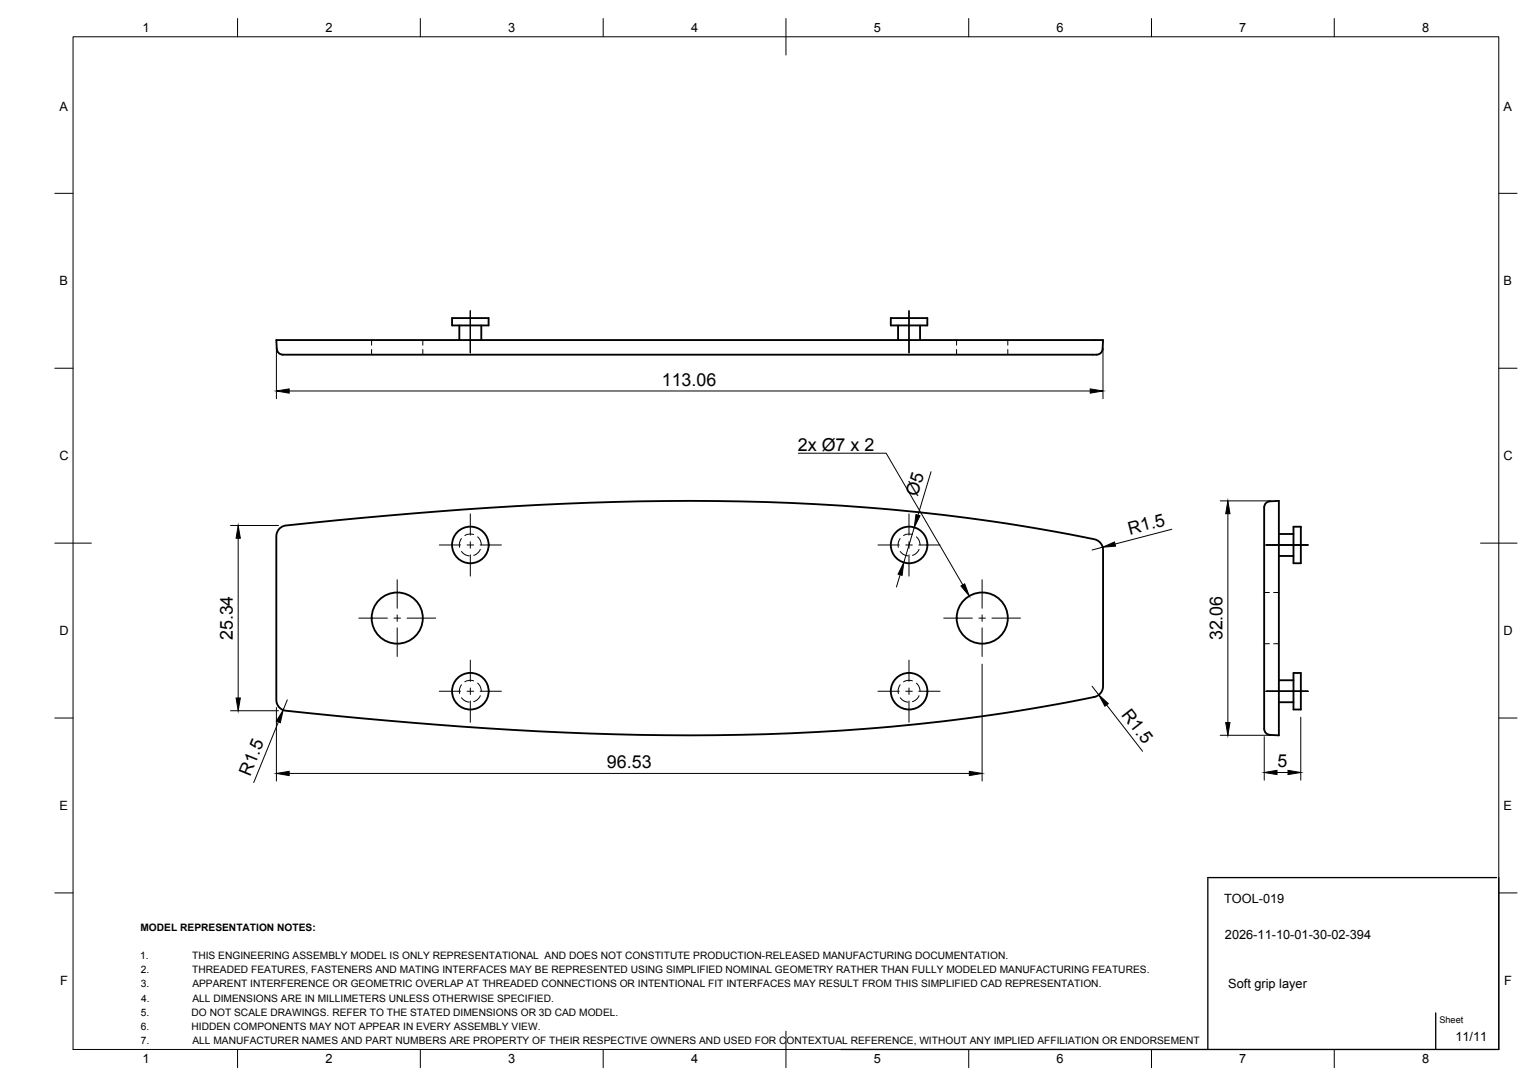
ISO-10303-21;
HEADER;
/* Generated by software containing ST-Developer
 * from STEP Tools, Inc. (www.steptools.com) 
 */

FILE_DESCRIPTION(
/* description */ (''),
/* implementation_level */ '2;1');

FILE_NAME(
/* name */ 'Soft grip layer.step',
/* time_stamp */ '2026-11-10T09:14:46-08:00',
/* author */ (''),
/* organization */ (''),
/* preprocessor_version */ 'ST-DEVELOPER v20.2',
/* originating_system */ 'Autodesk Translation Framework v15.17.0.0',
/* authorisation */ '');

FILE_SCHEMA (('AUTOMOTIVE_DESIGN { 1 0 10303 214 3 1 1 }'));
ENDSEC;

DATA;
#10=MECHANICAL_DESIGN_GEOMETRIC_PRESENTATION_REPRESENTATION('',(#564),#19471);
#156=B_SPLINE_SURFACE_WITH_KNOTS('',3,3,((#13811,#13812,#13813,#13814,#13815),
(#13816,#13817,#13818,#13819,#13820),(#13821,#13822,#13823,#13824,#13825),
(#13826,#13827,#13828,#13829,#13830),(#13831,#13832,#13833,#13834,#13835)),
 .UNSPECIFIED.,.F.,.F.,.F.,(4,1,4),(4,1,4),(0.,0.571428571428571,1.),(0.,
0.0439228984074713,0.102486762950766),.UNSPECIFIED.);
#157=B_SPLINE_SURFACE_WITH_KNOTS('',3,3,((#13858,#13859,#13860,#13861,#13862),
(#13863,#13864,#13865,#13866,#13867),(#13868,#13869,#13870,#13871,#13872),
(#13873,#13874,#13875,#13876,#13877),(#13878,#13879,#13880,#13881,#13882)),
 .UNSPECIFIED.,.F.,.F.,.F.,(4,1,4),(4,1,4),(0.,0.571428571428571,1.),(0.,
0.0439228984484775,0.102486763046448),.UNSPECIFIED.);
#158=B_SPLINE_SURFACE_WITH_KNOTS('',3,3,((#13896,#13897,#13898,#13899,#13900,
#13901),(#13902,#13903,#13904,#13905,#13906,#13907),(#13908,#13909,#13910,
#13911,#13912,#13913),(#13914,#13915,#13916,#13917,#13918,#13919),(#13920,
#13921,#13922,#13923,#13924,#13925)),.UNSPECIFIED.,.F.,.F.,.F.,(4,1,4),
(4,1,1,4),(0.,0.571428571428571,1.),(0.,4.74079765360458,7.9013294226743,
11.061861191744),.UNSPECIFIED.);
#159=B_SPLINE_SURFACE_WITH_KNOTS('',3,3,((#13941,#13942,#13943,#13944,#13945),
(#13946,#13947,#13948,#13949,#13950),(#13951,#13952,#13953,#13954,#13955),
(#13956,#13957,#13958,#13959,#13960),(#13961,#13962,#13963,#13964,#13965)),
 .UNSPECIFIED.,.F.,.F.,.F.,(4,1,4),(4,1,4),(0.,0.571428571428571,1.),(0.,
0.0409389169025732,0.0955241394393374),.UNSPECIFIED.);
#160=B_SPLINE_SURFACE_WITH_KNOTS('',3,3,((#13985,#13986,#13987,#13988,#13989),
(#13990,#13991,#13992,#13993,#13994),(#13995,#13996,#13997,#13998,#13999),
(#14000,#14001,#14002,#14003,#14004),(#14005,#14006,#14007,#14008,#14009)),
 .UNSPECIFIED.,.F.,.F.,.F.,(4,1,4),(4,1,4),(0.,0.571428571428571,1.),(2.31010434703409E-17,
0.054585222365383,0.0955241391394202),.UNSPECIFIED.);
#161=B_SPLINE_SURFACE_WITH_KNOTS('',3,3,((#14023,#14024,#14025,#14026,#14027,
#14028),(#14029,#14030,#14031,#14032,#14033,#14034),(#14035,#14036,#14037,
#14038,#14039,#14040),(#14041,#14042,#14043,#14044,#14045,#14046),(#14047,
#14048,#14049,#14050,#14051,#14052)),.UNSPECIFIED.,.F.,.F.,.F.,(4,1,4),
(4,1,1,4),(0.,0.571428571428571,1.),(1.48308270761676E-15,3.16052629084276,
6.32105258168553,11.0618420179497),.UNSPECIFIED.);
#162=B_SPLINE_SURFACE_WITH_KNOTS('',3,3,((#14077,#14078,#14079,#14080),
(#14081,#14082,#14083,#14084),(#14085,#14086,#14087,#14088),(#14089,#14090,
#14091,#14092),(#14093,#14094,#14095,#14096)),.UNSPECIFIED.,.F.,.F.,.F.,
(4,1,4),(4,4),(0.,0.571428571428571,1.),(-0.0018994230917637,0.12591792480537),
 .UNSPECIFIED.);
#163=B_SPLINE_SURFACE_WITH_KNOTS('',3,3,((#14127,#14128,#14129,#14130),
(#14131,#14132,#14133,#14134),(#14135,#14136,#14137,#14138),(#14139,#14140,
#14141,#14142)),.UNSPECIFIED.,.F.,.F.,.F.,(4,4),(4,4),(0.0105624938889701,
0.988135278219398),(0.,0.624639504152193),.UNSPECIFIED.);
#164=B_SPLINE_SURFACE_WITH_KNOTS('',3,3,((#14152,#14153,#14154,#14155),
(#14156,#14157,#14158,#14159),(#14160,#14161,#14162,#14163),(#14164,#14165,
#14166,#14167),(#14168,#14169,#14170,#14171)),.UNSPECIFIED.,.F.,.F.,.F.,
(4,1,4),(4,4),(0.,0.571428571428571,1.),(-0.00248141748936713,0.125282751535517),
 .UNSPECIFIED.);
#165=B_SPLINE_SURFACE_WITH_KNOTS('',3,3,((#14213,#14214,#14215,#14216),
(#14217,#14218,#14219,#14220),(#14221,#14222,#14223,#14224),(#14225,#14226,
#14227,#14228),(#14229,#14230,#14231,#14232)),.UNSPECIFIED.,.F.,.F.,.F.,
(4,1,4),(4,4),(0.,0.571428571428571,1.),(-0.00183337806924316,0.12591792480537),
 .UNSPECIFIED.);
#166=B_SPLINE_SURFACE_WITH_KNOTS('',3,3,((#14263,#14264,#14265,#14266),
(#14267,#14268,#14269,#14270),(#14271,#14272,#14273,#14274),(#14275,#14276,
#14277,#14278),(#14279,#14280,#14281,#14282)),.UNSPECIFIED.,.F.,.F.,.F.,
(4,1,4),(4,4),(0.,0.571428571428571,1.),(-0.00256306836558615,0.125282751535516),
 .UNSPECIFIED.);
#167=B_SPLINE_SURFACE_WITH_KNOTS('',3,3,((#14321,#14322,#14323,#14324),
(#14325,#14326,#14327,#14328),(#14329,#14330,#14331,#14332),(#14333,#14334,
#14335,#14336)),.UNSPECIFIED.,.F.,.F.,.F.,(4,4),(4,4),(0.0118647217806023,
0.98943750611103),(0.,0.624639504152185),.UNSPECIFIED.);
#356=B_SPLINE_CURVE_WITH_KNOTS('',3,(#13840,#13841,#13842,#13843,#13844),
 .UNSPECIFIED.,.F.,.F.,(4,1,4),(-0.102486762950766,-0.0439228984074713,
0.),.UNSPECIFIED.);
#357=B_SPLINE_CURVE_WITH_KNOTS('',3,(#13847,#13848,#13849,#13850,#13851),
 .UNSPECIFIED.,.F.,.F.,(4,1,4),(0.,0.0439228984074713,0.102486762950766),
 .UNSPECIFIED.);
#358=B_SPLINE_CURVE_WITH_KNOTS('',3,(#13886,#13887,#13888,#13889,#13890),
 .UNSPECIFIED.,.F.,.F.,(4,1,4),(-0.102486763046448,-0.0439228984484775,
0.),.UNSPECIFIED.);
#359=B_SPLINE_CURVE_WITH_KNOTS('',3,(#13891,#13892,#13893,#13894,#13895),
 .UNSPECIFIED.,.F.,.F.,(4,1,4),(0.,0.0439228984484775,0.102486763046448),
 .UNSPECIFIED.);
#360=B_SPLINE_CURVE_WITH_KNOTS('',3,(#13929,#13930,#13931,#13932,#13933,
#13934),.UNSPECIFIED.,.F.,.F.,(4,1,1,4),(-11.061861191744,-7.9013294226743,
-4.74079765360458,0.),.UNSPECIFIED.);
#361=B_SPLINE_CURVE_WITH_KNOTS('',3,(#13935,#13936,#13937,#13938,#13939,
#13940),.UNSPECIFIED.,.F.,.F.,(4,1,1,4),(0.,4.74079765360458,7.9013294226743,
11.061861191744),.UNSPECIFIED.);
#362=B_SPLINE_CURVE_WITH_KNOTS('',3,(#13969,#13970,#13971,#13972,#13973),
 .UNSPECIFIED.,.F.,.F.,(4,1,4),(-0.0955241394393374,-0.0409389169025732,
0.),.UNSPECIFIED.);
#363=B_SPLINE_CURVE_WITH_KNOTS('',3,(#13974,#13975,#13976,#13977,#13978),
 .UNSPECIFIED.,.F.,.F.,(4,1,4),(0.,0.0409389169025732,0.0955241394393374),
 .UNSPECIFIED.);
#364=B_SPLINE_CURVE_WITH_KNOTS('',3,(#14013,#14014,#14015,#14016,#14017),
 .UNSPECIFIED.,.F.,.F.,(4,1,4),(-0.0955241391394202,-0.054585222365383,
-2.31010434703409E-17),.UNSPECIFIED.);
#365=B_SPLINE_CURVE_WITH_KNOTS('',3,(#14018,#14019,#14020,#14021,#14022),
 .UNSPECIFIED.,.F.,.F.,(4,1,4),(2.31010434703409E-17,0.054585222365383,
0.0955241391394202),.UNSPECIFIED.);
#366=B_SPLINE_CURVE_WITH_KNOTS('',3,(#14053,#14054,#14055,#14056,#14057,
#14058),.UNSPECIFIED.,.F.,.F.,(4,1,1,4),(-11.0618420179497,-6.32105258168553,
-3.16052629084276,-1.48308270761676E-15),.UNSPECIFIED.);
#367=B_SPLINE_CURVE_WITH_KNOTS('',3,(#14059,#14060,#14061,#14062,#14063,
#14064),.UNSPECIFIED.,.F.,.F.,(4,1,1,4),(1.48308270761676E-15,3.16052629084276,
6.32105258168553,11.0618420179497),.UNSPECIFIED.);
#368=B_SPLINE_CURVE_WITH_KNOTS('',3,(#14067,#14068,#14069,#14070),
 .UNSPECIFIED.,.F.,.F.,(4,4),(0.00139191041679171,0.12591792480537),
 .UNSPECIFIED.);
#369=B_SPLINE_CURVE_WITH_KNOTS('',3,(#14073,#14074,#14075,#14076),
 .UNSPECIFIED.,.F.,.F.,(4,4),(-0.12591792480537,-0.00139191041679165),
 .UNSPECIFIED.);
#370=B_SPLINE_CURVE_WITH_KNOTS('',3,(#14098,#14099,#14100,#14101),
 .UNSPECIFIED.,.F.,.F.,(4,4),(-0.125267757839186,2.34187669256869E-17),
 .UNSPECIFIED.);
#371=B_SPLINE_CURVE_WITH_KNOTS('',3,(#14102,#14103,#14104,#14105,#14106,
#14107,#14108,#14109,#14110,#14111,#14112,#14113,#14114,#14115,#14116,#14117,
#14118,#14119,#14120,#14121,#14122,#14123,#14124,#14125,#14126),
 .UNSPECIFIED.,.F.,.F.,(4,3,3,3,3,3,3,3,4),(0.,0.0322618866145428,0.0585630993998112,
0.0880157356071287,0.11701919887454,0.14936655709923,0.161132799378038,
0.193259076308563,0.205272292311979),.UNSPECIFIED.);
#372=B_SPLINE_CURVE_WITH_KNOTS('',3,(#14144,#14145,#14146,#14147),
 .UNSPECIFIED.,.F.,.F.,(4,4),(-1.85615411929518E-16,0.12492953807382),
 .UNSPECIFIED.);
#373=B_SPLINE_CURVE_WITH_KNOTS('',3,(#14148,#14149,#14150,#14151),
 .UNSPECIFIED.,.F.,.F.,(4,4),(0.0105624938889701,0.988135278219398),
 .UNSPECIFIED.);
#374=B_SPLINE_CURVE_WITH_KNOTS('',3,(#14173,#14174,#14175,#14176),
 .UNSPECIFIED.,.F.,.F.,(4,4),(-0.125282751535517,-0.000756099764976127),
 .UNSPECIFIED.);
#375=B_SPLINE_CURVE_WITH_KNOTS('',3,(#14177,#14178,#14179,#14180,#14181,
#14182,#14183,#14184,#14185,#14186,#14187,#14188,#14189,#14190,#14191,#14192,
#14193,#14194,#14195,#14196,#14197,#14198,#14199,#14200,#14201,#14202,#14203,
#14204),.UNSPECIFIED.,.F.,.F.,(4,3,3,3,3,3,3,3,3,4),(0.,0.0322721186185131,
0.0586507621648183,0.090893271235385,0.0944607523249211,0.117149429440675,
0.149538018358679,0.168700492523839,0.200858914363656,0.220277485057336),
 .UNSPECIFIED.);
#376=B_SPLINE_CURVE_WITH_KNOTS('',3,(#14208,#14209,#14210,#14211),
 .UNSPECIFIED.,.F.,.F.,(4,4),(0.000756099764976051,0.125282751535516),
 .UNSPECIFIED.);
#377=B_SPLINE_CURVE_WITH_KNOTS('',3,(#14234,#14235,#14236,#14237,#14238,
#14239,#14240,#14241,#14242,#14243,#14244,#14245,#14246,#14247,#14248,#14249,
#14250,#14251,#14252,#14253,#14254,#14255,#14256,#14257,#14258),
 .UNSPECIFIED.,.F.,.F.,(4,3,3,3,3,3,3,3,4),(-1.38777878078145E-17,0.0322740250441291,
0.0586501551213245,0.0880475535304867,0.117148640042868,0.149495851515852,
0.161204029299056,0.193312734374797,0.205276387553207),.UNSPECIFIED.);
#378=B_SPLINE_CURVE_WITH_KNOTS('',3,(#14259,#14260,#14261,#14262),
 .UNSPECIFIED.,.F.,.F.,(4,4),(5.20417042793042E-18,0.125267757839184),
 .UNSPECIFIED.);
#379=B_SPLINE_CURVE_WITH_KNOTS('',3,(#14284,#14285,#14286,#14287),
 .UNSPECIFIED.,.F.,.F.,(4,4),(-0.124929538073804,-1.0547118733939E-15),
 .UNSPECIFIED.);
#380=B_SPLINE_CURVE_WITH_KNOTS('',3,(#14288,#14289,#14290,#14291,#14292,
#14293,#14294,#14295,#14296,#14297,#14298,#14299,#14300,#14301,#14302,#14303,
#14304,#14305,#14306,#14307,#14308,#14309,#14310,#14311,#14312,#14313,#14314,
#14315),.UNSPECIFIED.,.F.,.F.,(4,3,3,3,3,3,3,3,3,4),(0.,0.0322648940196546,
0.0586047006713273,0.0908498906869236,0.0944423330072586,0.117077542275299,
0.149464200283694,0.168660330271145,0.200827593216919,0.220275105166519),
 .UNSPECIFIED.);
#381=B_SPLINE_CURVE_WITH_KNOTS('',3,(#14317,#14318,#14319,#14320),
 .UNSPECIFIED.,.F.,.F.,(4,4),(0.0118647217806024,0.98943750611103),
 .UNSPECIFIED.);
#544=SHAPE_REPRESENTATION_RELATIONSHIP('SRR','None',#19524,#554);
#554=ADVANCED_BREP_SHAPE_REPRESENTATION('',(#574),#19467);
#564=STYLED_ITEM('',(#19585),#574);
#574=MANIFOLD_SOLID_BREP('Body1',#7157);
#635=FACE_BOUND('',#1556,.T.);
#636=FACE_BOUND('',#1560,.T.);
#637=FACE_BOUND('',#1564,.T.);
#638=FACE_BOUND('',#1568,.T.);
#639=FACE_BOUND('',#1588,.T.);
#640=FACE_BOUND('',#1589,.T.);
#641=FACE_BOUND('',#1594,.T.);
#642=FACE_BOUND('',#1595,.T.);
#643=FACE_BOUND('',#1596,.T.);
#644=FACE_BOUND('',#1597,.T.);
#645=FACE_BOUND('',#1598,.T.);
#646=FACE_BOUND('',#1599,.T.);
#788=PLANE('',#7640);
#789=PLANE('',#7645);
#790=PLANE('',#7646);
#791=PLANE('',#7651);
#792=PLANE('',#7652);
#793=PLANE('',#7657);
#794=PLANE('',#7658);
#795=PLANE('',#7663);
#796=PLANE('',#7682);
#797=PLANE('',#7683);
#798=PLANE('',#7684);
#799=PLANE('',#7685);
#1091=FACE_OUTER_BOUND('',#1553,.T.);
#1092=FACE_OUTER_BOUND('',#1554,.T.);
#1093=FACE_OUTER_BOUND('',#1555,.T.);
#1094=FACE_OUTER_BOUND('',#1557,.T.);
#1095=FACE_OUTER_BOUND('',#1558,.T.);
#1096=FACE_OUTER_BOUND('',#1559,.T.);
#1097=FACE_OUTER_BOUND('',#1561,.T.);
#1098=FACE_OUTER_BOUND('',#1562,.T.);
#1099=FACE_OUTER_BOUND('',#1563,.T.);
#1100=FACE_OUTER_BOUND('',#1565,.T.);
#1101=FACE_OUTER_BOUND('',#1566,.T.);
#1102=FACE_OUTER_BOUND('',#1567,.T.);
#1103=FACE_OUTER_BOUND('',#1569,.T.);
#1104=FACE_OUTER_BOUND('',#1570,.T.);
#1105=FACE_OUTER_BOUND('',#1571,.T.);
#1106=FACE_OUTER_BOUND('',#1572,.T.);
#1107=FACE_OUTER_BOUND('',#1573,.T.);
#1108=FACE_OUTER_BOUND('',#1574,.T.);
#1109=FACE_OUTER_BOUND('',#1575,.T.);
#1110=FACE_OUTER_BOUND('',#1576,.T.);
#1111=FACE_OUTER_BOUND('',#1577,.T.);
#1112=FACE_OUTER_BOUND('',#1578,.T.);
#1113=FACE_OUTER_BOUND('',#1579,.T.);
#1114=FACE_OUTER_BOUND('',#1580,.T.);
#1115=FACE_OUTER_BOUND('',#1581,.T.);
#1116=FACE_OUTER_BOUND('',#1582,.T.);
#1117=FACE_OUTER_BOUND('',#1583,.T.);
#1118=FACE_OUTER_BOUND('',#1584,.T.);
#1119=FACE_OUTER_BOUND('',#1585,.T.);
#1120=FACE_OUTER_BOUND('',#1586,.T.);
#1121=FACE_OUTER_BOUND('',#1587,.T.);
#1122=FACE_OUTER_BOUND('',#1590,.T.);
#1123=FACE_OUTER_BOUND('',#1591,.T.);
#1124=FACE_OUTER_BOUND('',#1592,.T.);
#1125=FACE_OUTER_BOUND('',#1593,.T.);
#1126=FACE_OUTER_BOUND('',#1600,.T.);
#1553=EDGE_LOOP('',(#5897,#5898,#5899,#5900));
#1554=EDGE_LOOP('',(#5901,#5902,#5903,#5904));
#1555=EDGE_LOOP('',(#5905));
#1556=EDGE_LOOP('',(#5906));
#1557=EDGE_LOOP('',(#5907,#5908,#5909,#5910));
#1558=EDGE_LOOP('',(#5911));
#1559=EDGE_LOOP('',(#5912));
#1560=EDGE_LOOP('',(#5913));
#1561=EDGE_LOOP('',(#5914,#5915,#5916,#5917));
#1562=EDGE_LOOP('',(#5918));
#1563=EDGE_LOOP('',(#5919));
#1564=EDGE_LOOP('',(#5920));
#1565=EDGE_LOOP('',(#5921,#5922,#5923,#5924));
#1566=EDGE_LOOP('',(#5925));
#1567=EDGE_LOOP('',(#5926));
#1568=EDGE_LOOP('',(#5927));
#1569=EDGE_LOOP('',(#5928,#5929,#5930,#5931));
#1570=EDGE_LOOP('',(#5932));
#1571=EDGE_LOOP('',(#5933,#5934,#5935,#5936));
#1572=EDGE_LOOP('',(#5937,#5938,#5939,#5940));
#1573=EDGE_LOOP('',(#5941,#5942,#5943,#5944));
#1574=EDGE_LOOP('',(#5945,#5946,#5947,#5948));
#1575=EDGE_LOOP('',(#5949,#5950,#5951,#5952));
#1576=EDGE_LOOP('',(#5953,#5954,#5955,#5956));
#1577=EDGE_LOOP('',(#5957,#5958,#5959,#5960));
#1578=EDGE_LOOP('',(#5961,#5962,#5963,#5964));
#1579=EDGE_LOOP('',(#5965,#5966,#5967,#5968));
#1580=EDGE_LOOP('',(#5969,#5970,#5971,#5972));
#1581=EDGE_LOOP('',(#5973,#5974,#5975,#5976));
#1582=EDGE_LOOP('',(#5977,#5978,#5979,#5980));
#1583=EDGE_LOOP('',(#5981,#5982,#5983,#5984));
#1584=EDGE_LOOP('',(#5985,#5986,#5987,#5988));
#1585=EDGE_LOOP('',(#5989,#5990,#5991,#5992));
#1586=EDGE_LOOP('',(#5993,#5994,#5995,#5996));
#1587=EDGE_LOOP('',(#5997,#5998,#5999,#6000,#6001,#6002,#6003,#6004));
#1588=EDGE_LOOP('',(#6005));
#1589=EDGE_LOOP('',(#6006));
#1590=EDGE_LOOP('',(#6007,#6008,#6009,#6010));
#1591=EDGE_LOOP('',(#6011,#6012,#6013,#6014));
#1592=EDGE_LOOP('',(#6015,#6016,#6017,#6018));
#1593=EDGE_LOOP('',(#6019,#6020,#6021,#6022,#6023,#6024,#6025,#6026));
#1594=EDGE_LOOP('',(#6027));
#1595=EDGE_LOOP('',(#6028));
#1596=EDGE_LOOP('',(#6029));
#1597=EDGE_LOOP('',(#6030));
#1598=EDGE_LOOP('',(#6031));
#1599=EDGE_LOOP('',(#6032));
#1600=EDGE_LOOP('',(#6033,#6034,#6035,#6036));
#2057=LINE('',#13747,#2531);
#2058=LINE('',#13753,#2532);
#2059=LINE('',#13763,#2533);
#2060=LINE('',#13773,#2534);
#2061=LINE('',#13783,#2535);
#2062=LINE('',#13793,#2536);
#2063=LINE('',#13797,#2537);
#2064=LINE('',#13801,#2538);
#2065=LINE('',#13805,#2539);
#2066=LINE('',#13809,#2540);
#2067=LINE('',#13856,#2541);
#2068=LINE('',#13857,#2542);
#2069=LINE('',#13983,#2543);
#2070=LINE('',#13984,#2544);
#2071=LINE('',#14072,#2545);
#2072=LINE('',#14212,#2546);
#2531=VECTOR('',#8895,0.35);
#2532=VECTOR('',#8902,0.35);
#2533=VECTOR('',#8915,0.25);
#2534=VECTOR('',#8928,0.25);
#2535=VECTOR('',#8941,0.25);
#2536=VECTOR('',#8954,0.25);
#2537=VECTOR('',#8959,0.15);
#2538=VECTOR('',#8964,0.15);
#2539=VECTOR('',#8969,0.15);
#2540=VECTOR('',#8974,0.15);
#2541=VECTOR('',#8985,1.);
#2542=VECTOR('',#8986,1.);
#2543=VECTOR('',#8997,1.);
#2544=VECTOR('',#8998,1.);
#2545=VECTOR('',#9003,1.);
#2546=VECTOR('',#9008,1.);
#2803=CIRCLE('',#7635,0.35);
#2804=CIRCLE('',#7636,0.35);
#2805=CIRCLE('',#7638,0.35);
#2806=CIRCLE('',#7639,0.35);
#2807=CIRCLE('',#7641,0.25);
#2808=CIRCLE('',#7642,0.15);
#2809=CIRCLE('',#7644,0.25);
#2810=CIRCLE('',#7647,0.25);
#2811=CIRCLE('',#7648,0.15);
#2812=CIRCLE('',#7650,0.25);
#2813=CIRCLE('',#7653,0.25);
#2814=CIRCLE('',#7654,0.15);
#2815=CIRCLE('',#7656,0.25);
#2816=CIRCLE('',#7659,0.25);
#2817=CIRCLE('',#7660,0.15);
#2818=CIRCLE('',#7662,0.25);
#2819=CIRCLE('',#7665,0.15);
#2820=CIRCLE('',#7667,0.15);
#2821=CIRCLE('',#7669,0.15);
#2822=CIRCLE('',#7671,0.15);
#2823=CIRCLE('',#7672,0.0800000000000001);
#2824=CIRCLE('',#7673,0.0799999999999999);
#2825=CIRCLE('',#7675,0.0800000000000001);
#2826=CIRCLE('',#7676,0.0799999999999998);
#2827=CIRCLE('',#7677,0.0800000000000001);
#2828=CIRCLE('',#7678,0.0800000000000001);
#2829=CIRCLE('',#7680,0.0800000000000001);
#2830=CIRCLE('',#7681,0.0799999999999998);
#3279=VERTEX_POINT('',#13744);
#3280=VERTEX_POINT('',#13746);
#3281=VERTEX_POINT('',#13750);
#3282=VERTEX_POINT('',#13752);
#3283=VERTEX_POINT('',#13756);
#3284=VERTEX_POINT('',#13758);
#3285=VERTEX_POINT('',#13761);
#3286=VERTEX_POINT('',#13766);
#3287=VERTEX_POINT('',#13768);
#3288=VERTEX_POINT('',#13771);
#3289=VERTEX_POINT('',#13776);
#3290=VERTEX_POINT('',#13778);
#3291=VERTEX_POINT('',#13781);
#3292=VERTEX_POINT('',#13786);
#3293=VERTEX_POINT('',#13788);
#3294=VERTEX_POINT('',#13791);
#3295=VERTEX_POINT('',#13796);
#3296=VERTEX_POINT('',#13800);
#3297=VERTEX_POINT('',#13804);
#3298=VERTEX_POINT('',#13808);
#3299=VERTEX_POINT('',#13836);
#3300=VERTEX_POINT('',#13837);
#3301=VERTEX_POINT('',#13839);
#3302=VERTEX_POINT('',#13845);
#3303=VERTEX_POINT('',#13853);
#3304=VERTEX_POINT('',#13854);
#3305=VERTEX_POINT('',#13883);
#3306=VERTEX_POINT('',#13884);
#3307=VERTEX_POINT('',#13926);
#3308=VERTEX_POINT('',#13927);
#3309=VERTEX_POINT('',#13966);
#3310=VERTEX_POINT('',#13967);
#3311=VERTEX_POINT('',#13980);
#3312=VERTEX_POINT('',#13981);
#3313=VERTEX_POINT('',#14010);
#3314=VERTEX_POINT('',#14011);
#3315=VERTEX_POINT('',#14066);
#3316=VERTEX_POINT('',#14071);
#3317=VERTEX_POINT('',#14097);
#3318=VERTEX_POINT('',#14143);
#3319=VERTEX_POINT('',#14172);
#3320=VERTEX_POINT('',#14207);
#3321=VERTEX_POINT('',#14233);
#3322=VERTEX_POINT('',#14283);
#4189=EDGE_CURVE('',#3279,#3279,#2803,.T.);
#4190=EDGE_CURVE('',#3279,#3280,#2057,.T.);
#4191=EDGE_CURVE('',#3280,#3280,#2804,.T.);
#4192=EDGE_CURVE('',#3281,#3281,#2805,.T.);
#4193=EDGE_CURVE('',#3281,#3282,#2058,.T.);
#4194=EDGE_CURVE('',#3282,#3282,#2806,.T.);
#4195=EDGE_CURVE('',#3283,#3283,#2807,.T.);
#4196=EDGE_CURVE('',#3284,#3284,#2808,.T.);
#4197=EDGE_CURVE('',#3285,#3285,#2809,.T.);
#4198=EDGE_CURVE('',#3285,#3283,#2059,.T.);
#4199=EDGE_CURVE('',#3286,#3286,#2810,.T.);
#4200=EDGE_CURVE('',#3287,#3287,#2811,.T.);
#4201=EDGE_CURVE('',#3288,#3288,#2812,.T.);
#4202=EDGE_CURVE('',#3288,#3286,#2060,.T.);
#4203=EDGE_CURVE('',#3289,#3289,#2813,.T.);
#4204=EDGE_CURVE('',#3290,#3290,#2814,.T.);
#4205=EDGE_CURVE('',#3291,#3291,#2815,.T.);
#4206=EDGE_CURVE('',#3291,#3289,#2061,.T.);
#4207=EDGE_CURVE('',#3292,#3292,#2816,.T.);
#4208=EDGE_CURVE('',#3293,#3293,#2817,.T.);
#4209=EDGE_CURVE('',#3294,#3294,#2818,.T.);
#4210=EDGE_CURVE('',#3294,#3292,#2062,.T.);
#4211=EDGE_CURVE('',#3284,#3295,#2063,.T.);
#4212=EDGE_CURVE('',#3295,#3295,#2819,.T.);
#4213=EDGE_CURVE('',#3287,#3296,#2064,.T.);
#4214=EDGE_CURVE('',#3296,#3296,#2820,.T.);
#4215=EDGE_CURVE('',#3290,#3297,#2065,.T.);
#4216=EDGE_CURVE('',#3297,#3297,#2821,.T.);
#4217=EDGE_CURVE('',#3293,#3298,#2066,.T.);
#4218=EDGE_CURVE('',#3298,#3298,#2822,.T.);
#4219=EDGE_CURVE('',#3299,#3300,#2823,.T.);
#4220=EDGE_CURVE('',#3300,#3301,#356,.T.);
#4221=EDGE_CURVE('',#3301,#3302,#2824,.T.);
#4222=EDGE_CURVE('',#3302,#3299,#357,.T.);
#4223=EDGE_CURVE('',#3303,#3304,#2825,.T.);
#4224=EDGE_CURVE('',#3304,#3300,#2067,.T.);
#4225=EDGE_CURVE('',#3299,#3303,#2068,.T.);
#4226=EDGE_CURVE('',#3305,#3306,#2826,.T.);
#4227=EDGE_CURVE('',#3306,#3304,#358,.T.);
#4228=EDGE_CURVE('',#3303,#3305,#359,.T.);
#4229=EDGE_CURVE('',#3307,#3308,#2827,.T.);
#4230=EDGE_CURVE('',#3308,#3306,#360,.T.);
#4231=EDGE_CURVE('',#3305,#3307,#361,.T.);
#4232=EDGE_CURVE('',#3309,#3310,#2828,.T.);
#4233=EDGE_CURVE('',#3310,#3308,#362,.T.);
#4234=EDGE_CURVE('',#3307,#3309,#363,.T.);
#4235=EDGE_CURVE('',#3311,#3312,#2829,.T.);
#4236=EDGE_CURVE('',#3312,#3310,#2069,.T.);
#4237=EDGE_CURVE('',#3309,#3311,#2070,.T.);
#4238=EDGE_CURVE('',#3313,#3314,#2830,.T.);
#4239=EDGE_CURVE('',#3314,#3312,#364,.T.);
#4240=EDGE_CURVE('',#3311,#3313,#365,.T.);
#4241=EDGE_CURVE('',#3301,#3314,#366,.T.);
#4242=EDGE_CURVE('',#3313,#3302,#367,.T.);
#4243=EDGE_CURVE('',#3315,#3312,#368,.T.);
#4244=EDGE_CURVE('',#3316,#3315,#2071,.T.);
#4245=EDGE_CURVE('',#3310,#3316,#369,.T.);
#4246=EDGE_CURVE('',#3314,#3317,#370,.T.);
#4247=EDGE_CURVE('',#3317,#3315,#371,.T.);
#4248=EDGE_CURVE('',#3318,#3301,#372,.T.);
#4249=EDGE_CURVE('',#3317,#3318,#373,.T.);
#4250=EDGE_CURVE('',#3300,#3319,#374,.T.);
#4251=EDGE_CURVE('',#3319,#3318,#375,.T.);
#4252=EDGE_CURVE('',#3320,#3304,#376,.T.);
#4253=EDGE_CURVE('',#3319,#3320,#2072,.T.);
#4254=EDGE_CURVE('',#3316,#3321,#377,.T.);
#4255=EDGE_CURVE('',#3321,#3308,#378,.T.);
#4256=EDGE_CURVE('',#3306,#3322,#379,.T.);
#4257=EDGE_CURVE('',#3322,#3320,#380,.T.);
#4258=EDGE_CURVE('',#3322,#3321,#381,.T.);
#5897=ORIENTED_EDGE('',*,*,#4189,.F.);
#5898=ORIENTED_EDGE('',*,*,#4190,.T.);
#5899=ORIENTED_EDGE('',*,*,#4191,.F.);
#5900=ORIENTED_EDGE('',*,*,#4190,.F.);
#5901=ORIENTED_EDGE('',*,*,#4192,.F.);
#5902=ORIENTED_EDGE('',*,*,#4193,.T.);
#5903=ORIENTED_EDGE('',*,*,#4194,.F.);
#5904=ORIENTED_EDGE('',*,*,#4193,.F.);
#5905=ORIENTED_EDGE('',*,*,#4195,.T.);
#5906=ORIENTED_EDGE('',*,*,#4196,.T.);
#5907=ORIENTED_EDGE('',*,*,#4197,.F.);
#5908=ORIENTED_EDGE('',*,*,#4198,.T.);
#5909=ORIENTED_EDGE('',*,*,#4195,.F.);
#5910=ORIENTED_EDGE('',*,*,#4198,.F.);
#5911=ORIENTED_EDGE('',*,*,#4197,.T.);
#5912=ORIENTED_EDGE('',*,*,#4199,.T.);
#5913=ORIENTED_EDGE('',*,*,#4200,.T.);
#5914=ORIENTED_EDGE('',*,*,#4201,.F.);
#5915=ORIENTED_EDGE('',*,*,#4202,.T.);
#5916=ORIENTED_EDGE('',*,*,#4199,.F.);
#5917=ORIENTED_EDGE('',*,*,#4202,.F.);
#5918=ORIENTED_EDGE('',*,*,#4201,.T.);
#5919=ORIENTED_EDGE('',*,*,#4203,.T.);
#5920=ORIENTED_EDGE('',*,*,#4204,.T.);
#5921=ORIENTED_EDGE('',*,*,#4205,.F.);
#5922=ORIENTED_EDGE('',*,*,#4206,.T.);
#5923=ORIENTED_EDGE('',*,*,#4203,.F.);
#5924=ORIENTED_EDGE('',*,*,#4206,.F.);
#5925=ORIENTED_EDGE('',*,*,#4205,.T.);
#5926=ORIENTED_EDGE('',*,*,#4207,.T.);
#5927=ORIENTED_EDGE('',*,*,#4208,.T.);
#5928=ORIENTED_EDGE('',*,*,#4209,.F.);
#5929=ORIENTED_EDGE('',*,*,#4210,.T.);
#5930=ORIENTED_EDGE('',*,*,#4207,.F.);
#5931=ORIENTED_EDGE('',*,*,#4210,.F.);
#5932=ORIENTED_EDGE('',*,*,#4209,.T.);
#5933=ORIENTED_EDGE('',*,*,#4196,.F.);
#5934=ORIENTED_EDGE('',*,*,#4211,.T.);
#5935=ORIENTED_EDGE('',*,*,#4212,.F.);
#5936=ORIENTED_EDGE('',*,*,#4211,.F.);
#5937=ORIENTED_EDGE('',*,*,#4200,.F.);
#5938=ORIENTED_EDGE('',*,*,#4213,.T.);
#5939=ORIENTED_EDGE('',*,*,#4214,.F.);
#5940=ORIENTED_EDGE('',*,*,#4213,.F.);
#5941=ORIENTED_EDGE('',*,*,#4204,.F.);
#5942=ORIENTED_EDGE('',*,*,#4215,.T.);
#5943=ORIENTED_EDGE('',*,*,#4216,.F.);
#5944=ORIENTED_EDGE('',*,*,#4215,.F.);
#5945=ORIENTED_EDGE('',*,*,#4208,.F.);
#5946=ORIENTED_EDGE('',*,*,#4217,.T.);
#5947=ORIENTED_EDGE('',*,*,#4218,.F.);
#5948=ORIENTED_EDGE('',*,*,#4217,.F.);
#5949=ORIENTED_EDGE('',*,*,#4219,.T.);
#5950=ORIENTED_EDGE('',*,*,#4220,.T.);
#5951=ORIENTED_EDGE('',*,*,#4221,.T.);
#5952=ORIENTED_EDGE('',*,*,#4222,.T.);
#5953=ORIENTED_EDGE('',*,*,#4223,.T.);
#5954=ORIENTED_EDGE('',*,*,#4224,.T.);
#5955=ORIENTED_EDGE('',*,*,#4219,.F.);
#5956=ORIENTED_EDGE('',*,*,#4225,.T.);
#5957=ORIENTED_EDGE('',*,*,#4226,.T.);
#5958=ORIENTED_EDGE('',*,*,#4227,.T.);
#5959=ORIENTED_EDGE('',*,*,#4223,.F.);
#5960=ORIENTED_EDGE('',*,*,#4228,.T.);
#5961=ORIENTED_EDGE('',*,*,#4229,.T.);
#5962=ORIENTED_EDGE('',*,*,#4230,.T.);
#5963=ORIENTED_EDGE('',*,*,#4226,.F.);
#5964=ORIENTED_EDGE('',*,*,#4231,.T.);
#5965=ORIENTED_EDGE('',*,*,#4232,.T.);
#5966=ORIENTED_EDGE('',*,*,#4233,.T.);
#5967=ORIENTED_EDGE('',*,*,#4229,.F.);
#5968=ORIENTED_EDGE('',*,*,#4234,.T.);
#5969=ORIENTED_EDGE('',*,*,#4235,.T.);
#5970=ORIENTED_EDGE('',*,*,#4236,.T.);
#5971=ORIENTED_EDGE('',*,*,#4232,.F.);
#5972=ORIENTED_EDGE('',*,*,#4237,.T.);
#5973=ORIENTED_EDGE('',*,*,#4238,.T.);
#5974=ORIENTED_EDGE('',*,*,#4239,.T.);
#5975=ORIENTED_EDGE('',*,*,#4235,.F.);
#5976=ORIENTED_EDGE('',*,*,#4240,.T.);
#5977=ORIENTED_EDGE('',*,*,#4221,.F.);
#5978=ORIENTED_EDGE('',*,*,#4241,.T.);
#5979=ORIENTED_EDGE('',*,*,#4238,.F.);
#5980=ORIENTED_EDGE('',*,*,#4242,.T.);
#5981=ORIENTED_EDGE('',*,*,#4236,.F.);
#5982=ORIENTED_EDGE('',*,*,#4243,.F.);
#5983=ORIENTED_EDGE('',*,*,#4244,.F.);
#5984=ORIENTED_EDGE('',*,*,#4245,.F.);
#5985=ORIENTED_EDGE('',*,*,#4239,.F.);
#5986=ORIENTED_EDGE('',*,*,#4246,.T.);
#5987=ORIENTED_EDGE('',*,*,#4247,.T.);
#5988=ORIENTED_EDGE('',*,*,#4243,.T.);
#5989=ORIENTED_EDGE('',*,*,#4241,.F.);
#5990=ORIENTED_EDGE('',*,*,#4248,.F.);
#5991=ORIENTED_EDGE('',*,*,#4249,.F.);
#5992=ORIENTED_EDGE('',*,*,#4246,.F.);
#5993=ORIENTED_EDGE('',*,*,#4220,.F.);
#5994=ORIENTED_EDGE('',*,*,#4250,.T.);
#5995=ORIENTED_EDGE('',*,*,#4251,.T.);
#5996=ORIENTED_EDGE('',*,*,#4248,.T.);
#5997=ORIENTED_EDGE('',*,*,#4222,.F.);
#5998=ORIENTED_EDGE('',*,*,#4242,.F.);
#5999=ORIENTED_EDGE('',*,*,#4240,.F.);
#6000=ORIENTED_EDGE('',*,*,#4237,.F.);
#6001=ORIENTED_EDGE('',*,*,#4234,.F.);
#6002=ORIENTED_EDGE('',*,*,#4231,.F.);
#6003=ORIENTED_EDGE('',*,*,#4228,.F.);
#6004=ORIENTED_EDGE('',*,*,#4225,.F.);
#6005=ORIENTED_EDGE('',*,*,#4189,.T.);
#6006=ORIENTED_EDGE('',*,*,#4192,.T.);
#6007=ORIENTED_EDGE('',*,*,#4224,.F.);
#6008=ORIENTED_EDGE('',*,*,#4252,.F.);
#6009=ORIENTED_EDGE('',*,*,#4253,.F.);
#6010=ORIENTED_EDGE('',*,*,#4250,.F.);
#6011=ORIENTED_EDGE('',*,*,#4233,.F.);
#6012=ORIENTED_EDGE('',*,*,#4245,.T.);
#6013=ORIENTED_EDGE('',*,*,#4254,.T.);
#6014=ORIENTED_EDGE('',*,*,#4255,.T.);
#6015=ORIENTED_EDGE('',*,*,#4227,.F.);
#6016=ORIENTED_EDGE('',*,*,#4256,.T.);
#6017=ORIENTED_EDGE('',*,*,#4257,.T.);
#6018=ORIENTED_EDGE('',*,*,#4252,.T.);
#6019=ORIENTED_EDGE('',*,*,#4251,.F.);
#6020=ORIENTED_EDGE('',*,*,#4253,.T.);
#6021=ORIENTED_EDGE('',*,*,#4257,.F.);
#6022=ORIENTED_EDGE('',*,*,#4258,.T.);
#6023=ORIENTED_EDGE('',*,*,#4254,.F.);
#6024=ORIENTED_EDGE('',*,*,#4244,.T.);
#6025=ORIENTED_EDGE('',*,*,#4247,.F.);
#6026=ORIENTED_EDGE('',*,*,#4249,.T.);
#6027=ORIENTED_EDGE('',*,*,#4191,.T.);
#6028=ORIENTED_EDGE('',*,*,#4194,.T.);
#6029=ORIENTED_EDGE('',*,*,#4212,.T.);
#6030=ORIENTED_EDGE('',*,*,#4214,.T.);
#6031=ORIENTED_EDGE('',*,*,#4216,.T.);
#6032=ORIENTED_EDGE('',*,*,#4218,.T.);
#6033=ORIENTED_EDGE('',*,*,#4230,.F.);
#6034=ORIENTED_EDGE('',*,*,#4255,.F.);
#6035=ORIENTED_EDGE('',*,*,#4258,.F.);
#6036=ORIENTED_EDGE('',*,*,#4256,.F.);
#6653=CYLINDRICAL_SURFACE('',#7634,0.35);
#6654=CYLINDRICAL_SURFACE('',#7637,0.35);
#6655=CYLINDRICAL_SURFACE('',#7643,0.25);
#6656=CYLINDRICAL_SURFACE('',#7649,0.25);
#6657=CYLINDRICAL_SURFACE('',#7655,0.25);
#6658=CYLINDRICAL_SURFACE('',#7661,0.25);
#6659=CYLINDRICAL_SURFACE('',#7664,0.15);
#6660=CYLINDRICAL_SURFACE('',#7666,0.15);
#6661=CYLINDRICAL_SURFACE('',#7668,0.15);
#6662=CYLINDRICAL_SURFACE('',#7670,0.15);
#6663=CYLINDRICAL_SURFACE('',#7674,0.08);
#6664=CYLINDRICAL_SURFACE('',#7679,0.08);
#7013=ADVANCED_FACE('',(#1091),#6653,.F.);
#7014=ADVANCED_FACE('',(#1092),#6654,.F.);
#7015=ADVANCED_FACE('',(#1093,#635),#788,.T.);
#7016=ADVANCED_FACE('',(#1094),#6655,.T.);
#7017=ADVANCED_FACE('',(#1095),#789,.F.);
#7018=ADVANCED_FACE('',(#1096,#636),#790,.T.);
#7019=ADVANCED_FACE('',(#1097),#6656,.T.);
#7020=ADVANCED_FACE('',(#1098),#791,.F.);
#7021=ADVANCED_FACE('',(#1099,#637),#792,.T.);
#7022=ADVANCED_FACE('',(#1100),#6657,.T.);
#7023=ADVANCED_FACE('',(#1101),#793,.F.);
#7024=ADVANCED_FACE('',(#1102,#638),#794,.T.);
#7025=ADVANCED_FACE('',(#1103),#6658,.T.);
#7026=ADVANCED_FACE('',(#1104),#795,.F.);
#7027=ADVANCED_FACE('',(#1105),#6659,.T.);
#7028=ADVANCED_FACE('',(#1106),#6660,.T.);
#7029=ADVANCED_FACE('',(#1107),#6661,.T.);
#7030=ADVANCED_FACE('',(#1108),#6662,.T.);
#7031=ADVANCED_FACE('',(#1109),#156,.F.);
#7032=ADVANCED_FACE('',(#1110),#6663,.T.);
#7033=ADVANCED_FACE('',(#1111),#157,.F.);
#7034=ADVANCED_FACE('',(#1112),#158,.F.);
#7035=ADVANCED_FACE('',(#1113),#159,.F.);
#7036=ADVANCED_FACE('',(#1114),#6664,.T.);
#7037=ADVANCED_FACE('',(#1115),#160,.F.);
#7038=ADVANCED_FACE('',(#1116),#161,.F.);
#7039=ADVANCED_FACE('',(#1117),#796,.F.);
#7040=ADVANCED_FACE('',(#1118),#162,.F.);
#7041=ADVANCED_FACE('',(#1119),#163,.F.);
#7042=ADVANCED_FACE('',(#1120),#164,.F.);
#7043=ADVANCED_FACE('',(#1121,#639,#640),#797,.T.);
#7044=ADVANCED_FACE('',(#1122),#798,.F.);
#7045=ADVANCED_FACE('',(#1123),#165,.F.);
#7046=ADVANCED_FACE('',(#1124),#166,.F.);
#7047=ADVANCED_FACE('',(#1125,#641,#642,#643,#644,#645,#646),#799,.F.);
#7048=ADVANCED_FACE('',(#1126),#167,.F.);
#7157=CLOSED_SHELL('',(#7013,#7014,#7015,#7016,#7017,#7018,#7019,#7020,
#7021,#7022,#7023,#7024,#7025,#7026,#7027,#7028,#7029,#7030,#7031,#7032,
#7033,#7034,#7035,#7036,#7037,#7038,#7039,#7040,#7041,#7042,#7043,#7044,
#7045,#7046,#7047,#7048));
#7633=AXIS2_PLACEMENT_3D('',#13742,#8889,#8890);
#7634=AXIS2_PLACEMENT_3D('',#13743,#8891,#8892);
#7635=AXIS2_PLACEMENT_3D('',#13745,#8893,#8894);
#7636=AXIS2_PLACEMENT_3D('',#13748,#8896,#8897);
#7637=AXIS2_PLACEMENT_3D('',#13749,#8898,#8899);
#7638=AXIS2_PLACEMENT_3D('',#13751,#8900,#8901);
#7639=AXIS2_PLACEMENT_3D('',#13754,#8903,#8904);
#7640=AXIS2_PLACEMENT_3D('',#13755,#8905,#8906);
#7641=AXIS2_PLACEMENT_3D('',#13757,#8907,#8908);
#7642=AXIS2_PLACEMENT_3D('',#13759,#8909,#8910);
#7643=AXIS2_PLACEMENT_3D('',#13760,#8911,#8912);
#7644=AXIS2_PLACEMENT_3D('',#13762,#8913,#8914);
#7645=AXIS2_PLACEMENT_3D('',#13764,#8916,#8917);
#7646=AXIS2_PLACEMENT_3D('',#13765,#8918,#8919);
#7647=AXIS2_PLACEMENT_3D('',#13767,#8920,#8921);
#7648=AXIS2_PLACEMENT_3D('',#13769,#8922,#8923);
#7649=AXIS2_PLACEMENT_3D('',#13770,#8924,#8925);
#7650=AXIS2_PLACEMENT_3D('',#13772,#8926,#8927);
#7651=AXIS2_PLACEMENT_3D('',#13774,#8929,#8930);
#7652=AXIS2_PLACEMENT_3D('',#13775,#8931,#8932);
#7653=AXIS2_PLACEMENT_3D('',#13777,#8933,#8934);
#7654=AXIS2_PLACEMENT_3D('',#13779,#8935,#8936);
#7655=AXIS2_PLACEMENT_3D('',#13780,#8937,#8938);
#7656=AXIS2_PLACEMENT_3D('',#13782,#8939,#8940);
#7657=AXIS2_PLACEMENT_3D('',#13784,#8942,#8943);
#7658=AXIS2_PLACEMENT_3D('',#13785,#8944,#8945);
#7659=AXIS2_PLACEMENT_3D('',#13787,#8946,#8947);
#7660=AXIS2_PLACEMENT_3D('',#13789,#8948,#8949);
#7661=AXIS2_PLACEMENT_3D('',#13790,#8950,#8951);
#7662=AXIS2_PLACEMENT_3D('',#13792,#8952,#8953);
#7663=AXIS2_PLACEMENT_3D('',#13794,#8955,#8956);
#7664=AXIS2_PLACEMENT_3D('',#13795,#8957,#8958);
#7665=AXIS2_PLACEMENT_3D('',#13798,#8960,#8961);
#7666=AXIS2_PLACEMENT_3D('',#13799,#8962,#8963);
#7667=AXIS2_PLACEMENT_3D('',#13802,#8965,#8966);
#7668=AXIS2_PLACEMENT_3D('',#13803,#8967,#8968);
#7669=AXIS2_PLACEMENT_3D('',#13806,#8970,#8971);
#7670=AXIS2_PLACEMENT_3D('',#13807,#8972,#8973);
#7671=AXIS2_PLACEMENT_3D('',#13810,#8975,#8976);
#7672=AXIS2_PLACEMENT_3D('',#13838,#8977,#8978);
#7673=AXIS2_PLACEMENT_3D('',#13846,#8979,#8980);
#7674=AXIS2_PLACEMENT_3D('',#13852,#8981,#8982);
#7675=AXIS2_PLACEMENT_3D('',#13855,#8983,#8984);
#7676=AXIS2_PLACEMENT_3D('',#13885,#8987,#8988);
#7677=AXIS2_PLACEMENT_3D('',#13928,#8989,#8990);
#7678=AXIS2_PLACEMENT_3D('',#13968,#8991,#8992);
#7679=AXIS2_PLACEMENT_3D('',#13979,#8993,#8994);
#7680=AXIS2_PLACEMENT_3D('',#13982,#8995,#8996);
#7681=AXIS2_PLACEMENT_3D('',#14012,#8999,#9000);
#7682=AXIS2_PLACEMENT_3D('',#14065,#9001,#9002);
#7683=AXIS2_PLACEMENT_3D('',#14205,#9004,#9005);
#7684=AXIS2_PLACEMENT_3D('',#14206,#9006,#9007);
#7685=AXIS2_PLACEMENT_3D('',#14316,#9009,#9010);
#8889=DIRECTION('axis',(0.,0.,1.));
#8890=DIRECTION('refdir',(1.,0.,0.));
#8891=DIRECTION('center_axis',(0.,0.,-1.));
#8892=DIRECTION('ref_axis',(1.,0.,0.));
#8893=DIRECTION('center_axis',(-2.77374560774598E-32,-4.07593403759339E-32,
-1.));
#8894=DIRECTION('ref_axis',(1.,0.,0.));
#8895=DIRECTION('',(0.,0.,-1.));
#8896=DIRECTION('center_axis',(-3.68477953769876E-32,1.85992248306542E-19,
1.));
#8897=DIRECTION('ref_axis',(1.,0.,0.));
#8898=DIRECTION('center_axis',(0.,0.,-1.));
#8899=DIRECTION('ref_axis',(1.,0.,0.));
#8900=DIRECTION('center_axis',(-2.77374560774598E-32,-4.07593403759339E-32,
-1.));
#8901=DIRECTION('ref_axis',(1.,0.,0.));
#8902=DIRECTION('',(0.,0.,-1.));
#8903=DIRECTION('center_axis',(-3.68477953769876E-32,1.85992248306542E-19,
1.));
#8904=DIRECTION('ref_axis',(1.,0.,0.));
#8905=DIRECTION('center_axis',(0.,0.,1.));
#8906=DIRECTION('ref_axis',(1.,0.,0.));
#8907=DIRECTION('center_axis',(0.,0.,1.));
#8908=DIRECTION('ref_axis',(1.,0.,0.));
#8909=DIRECTION('center_axis',(0.,0.,-1.));
#8910=DIRECTION('ref_axis',(1.,0.,0.));
#8911=DIRECTION('center_axis',(0.,0.,-1.));
#8912=DIRECTION('ref_axis',(1.,0.,0.));
#8913=DIRECTION('center_axis',(0.,0.,-1.));
#8914=DIRECTION('ref_axis',(1.,0.,0.));
#8915=DIRECTION('',(0.,0.,1.));
#8916=DIRECTION('center_axis',(0.,0.,1.));
#8917=DIRECTION('ref_axis',(1.,0.,0.));
#8918=DIRECTION('center_axis',(0.,0.,1.));
#8919=DIRECTION('ref_axis',(1.,0.,0.));
#8920=DIRECTION('center_axis',(0.,0.,1.));
#8921=DIRECTION('ref_axis',(1.,0.,0.));
#8922=DIRECTION('center_axis',(0.,0.,-1.));
#8923=DIRECTION('ref_axis',(1.,0.,0.));
#8924=DIRECTION('center_axis',(0.,0.,-1.));
#8925=DIRECTION('ref_axis',(1.,0.,0.));
#8926=DIRECTION('center_axis',(0.,0.,-1.));
#8927=DIRECTION('ref_axis',(1.,0.,0.));
#8928=DIRECTION('',(0.,0.,1.));
#8929=DIRECTION('center_axis',(0.,0.,1.));
#8930=DIRECTION('ref_axis',(1.,0.,0.));
#8931=DIRECTION('center_axis',(0.,0.,1.));
#8932=DIRECTION('ref_axis',(1.,0.,0.));
#8933=DIRECTION('center_axis',(0.,0.,1.));
#8934=DIRECTION('ref_axis',(1.,0.,0.));
#8935=DIRECTION('center_axis',(0.,0.,-1.));
#8936=DIRECTION('ref_axis',(1.,0.,0.));
#8937=DIRECTION('center_axis',(0.,0.,-1.));
#8938=DIRECTION('ref_axis',(1.,0.,0.));
#8939=DIRECTION('center_axis',(0.,0.,-1.));
#8940=DIRECTION('ref_axis',(1.,0.,0.));
#8941=DIRECTION('',(0.,0.,1.));
#8942=DIRECTION('center_axis',(0.,0.,1.));
#8943=DIRECTION('ref_axis',(1.,0.,0.));
#8944=DIRECTION('center_axis',(0.,0.,1.));
#8945=DIRECTION('ref_axis',(1.,0.,0.));
#8946=DIRECTION('center_axis',(0.,0.,1.));
#8947=DIRECTION('ref_axis',(1.,0.,0.));
#8948=DIRECTION('center_axis',(0.,0.,-1.));
#8949=DIRECTION('ref_axis',(1.,0.,0.));
#8950=DIRECTION('center_axis',(0.,0.,-1.));
#8951=DIRECTION('ref_axis',(1.,0.,0.));
#8952=DIRECTION('center_axis',(0.,0.,-1.));
#8953=DIRECTION('ref_axis',(1.,0.,0.));
#8954=DIRECTION('',(0.,0.,1.));
#8955=DIRECTION('center_axis',(0.,0.,1.));
#8956=DIRECTION('ref_axis',(1.,0.,0.));
#8957=DIRECTION('center_axis',(0.,0.,-1.));
#8958=DIRECTION('ref_axis',(1.,0.,0.));
#8959=DIRECTION('',(0.,0.,1.));
#8960=DIRECTION('center_axis',(-3.68477953769876E-32,1.85992248306542E-19,
1.));
#8961=DIRECTION('ref_axis',(1.,0.,0.));
#8962=DIRECTION('center_axis',(0.,0.,-1.));
#8963=DIRECTION('ref_axis',(1.,0.,0.));
#8964=DIRECTION('',(0.,0.,1.));
#8965=DIRECTION('center_axis',(-3.68477953769876E-32,1.85992248306542E-19,
1.));
#8966=DIRECTION('ref_axis',(1.,0.,0.));
#8967=DIRECTION('center_axis',(0.,0.,-1.));
#8968=DIRECTION('ref_axis',(1.,0.,0.));
#8969=DIRECTION('',(0.,0.,1.));
#8970=DIRECTION('center_axis',(-3.68477953769876E-32,1.85992248306542E-19,
1.));
#8971=DIRECTION('ref_axis',(1.,0.,0.));
#8972=DIRECTION('center_axis',(0.,0.,-1.));
#8973=DIRECTION('ref_axis',(1.,0.,0.));
#8974=DIRECTION('',(0.,0.,1.));
#8975=DIRECTION('center_axis',(-3.68477953769876E-32,1.85992248306542E-19,
1.));
#8976=DIRECTION('ref_axis',(1.,0.,0.));
#8977=DIRECTION('center_axis',(0.,1.,0.));
#8978=DIRECTION('ref_axis',(0.,0.,1.));
#8979=DIRECTION('center_axis',(0.994535543241646,-0.104398530780106,0.));
#8980=DIRECTION('ref_axis',(0.104226596285684,0.992897637377125,0.0573680949450512));
#8981=DIRECTION('center_axis',(-2.13610651414414E-33,-1.,4.07593403759339E-32));
#8982=DIRECTION('ref_axis',(0.688354575693766,0.,0.725374371012276));
#8983=DIRECTION('center_axis',(0.,1.,0.));
#8984=DIRECTION('ref_axis',(0.,0.,1.));
#8985=DIRECTION('',(2.13610651414414E-33,1.,-4.07593403759339E-32));
#8986=DIRECTION('',(-2.13610651414414E-33,-1.,4.07593403759339E-32));
#8987=DIRECTION('center_axis',(0.994535543241646,0.104398530780106,0.));
#8988=DIRECTION('ref_axis',(0.,0.,1.));
#8989=DIRECTION('center_axis',(0.979252793246429,-0.20264246079997,0.));
#8990=DIRECTION('ref_axis',(0.,0.,1.));
#8991=DIRECTION('center_axis',(0.,-1.,0.));
#8992=DIRECTION('ref_axis',(-2.77555756156289E-15,0.,1.));
#8993=DIRECTION('center_axis',(-2.13610651414429E-33,1.,-4.07593403759339E-32));
#8994=DIRECTION('ref_axis',(-0.688354575693754,0.,0.725374371012288));
#8995=DIRECTION('center_axis',(0.,-1.,0.));
#8996=DIRECTION('ref_axis',(0.,0.,1.));
#8997=DIRECTION('',(2.13610651414429E-33,-1.,4.07593403759339E-32));
#8998=DIRECTION('',(-2.13610651414429E-33,1.,-4.07593403759339E-32));
#8999=DIRECTION('center_axis',(-0.979252793246429,-0.20264246079997,-4.07695874246507E-15));
#9000=DIRECTION('ref_axis',(-4.16333634234434E-15,0.,1.));
#9001=DIRECTION('center_axis',(0.998629534754574,0.,-0.0523359562429439));
#9002=DIRECTION('ref_axis',(-0.0523359562429439,0.,-0.998629534754574));
#9003=DIRECTION('',(0.,1.,0.));
#9004=DIRECTION('center_axis',(2.77374560774598E-32,4.07593403759339E-32,
1.));
#9005=DIRECTION('ref_axis',(1.,0.,-2.77374560774598E-32));
#9006=DIRECTION('center_axis',(-0.998629534754574,0.,-0.0523359562429402));
#9007=DIRECTION('ref_axis',(-0.0523359562429402,0.,0.998629534754574));
#9008=DIRECTION('',(0.,-1.,0.));
#9009=DIRECTION('center_axis',(-3.68477953769876E-32,1.85992248306542E-19,
1.));
#9010=DIRECTION('ref_axis',(1.,0.,3.68477953769876E-32));
#13742=CARTESIAN_POINT('',(0.,0.,0.));
#13743=CARTESIAN_POINT('Origin',(2.,0.,1.));
#13744=CARTESIAN_POINT('',(1.65,4.28626379701574E-17,1.1));
#13745=CARTESIAN_POINT('Origin',(2.,0.,1.1));
#13746=CARTESIAN_POINT('',(1.65,4.28626379701574E-17,0.9));
#13747=CARTESIAN_POINT('',(1.65,4.28626379701574E-17,1.));
#13748=CARTESIAN_POINT('Origin',(2.,0.,0.9));
#13749=CARTESIAN_POINT('Origin',(10.,0.,1.));
#13750=CARTESIAN_POINT('',(9.65,4.28626379701574E-17,1.1));
#13751=CARTESIAN_POINT('Origin',(10.,0.,1.1));
#13752=CARTESIAN_POINT('',(9.65,4.28626379701574E-17,0.9));
#13753=CARTESIAN_POINT('',(9.65,4.28626379701574E-17,1.));
#13754=CARTESIAN_POINT('Origin',(10.,0.,0.9));
#13755=CARTESIAN_POINT('Origin',(9.,1.,0.7));
#13756=CARTESIAN_POINT('',(8.75,1.,0.7));
#13757=CARTESIAN_POINT('Origin',(9.,1.,0.7));
#13758=CARTESIAN_POINT('',(8.85,1.,0.7));
#13759=CARTESIAN_POINT('Origin',(9.,1.,0.7));
#13760=CARTESIAN_POINT('Origin',(9.,1.,0.7));
#13761=CARTESIAN_POINT('',(8.75,1.,0.6));
#13762=CARTESIAN_POINT('Origin',(9.,1.,0.6));
#13763=CARTESIAN_POINT('',(8.75,1.,0.7));
#13764=CARTESIAN_POINT('Origin',(9.,1.,0.6));
#13765=CARTESIAN_POINT('Origin',(3.,-1.,0.7));
#13766=CARTESIAN_POINT('',(2.75,-1.,0.7));
#13767=CARTESIAN_POINT('Origin',(3.,-1.,0.7));
#13768=CARTESIAN_POINT('',(2.85,-1.,0.7));
#13769=CARTESIAN_POINT('Origin',(3.,-1.,0.7));
#13770=CARTESIAN_POINT('Origin',(3.,-1.,0.7));
#13771=CARTESIAN_POINT('',(2.75,-1.,0.6));
#13772=CARTESIAN_POINT('Origin',(3.,-1.,0.6));
#13773=CARTESIAN_POINT('',(2.75,-1.,0.7));
#13774=CARTESIAN_POINT('Origin',(3.,-1.,0.6));
#13775=CARTESIAN_POINT('Origin',(3.,1.,0.7));
#13776=CARTESIAN_POINT('',(2.75,1.,0.7));
#13777=CARTESIAN_POINT('Origin',(3.,1.,0.7));
#13778=CARTESIAN_POINT('',(2.85,1.,0.7));
#13779=CARTESIAN_POINT('Origin',(3.,1.,0.7));
#13780=CARTESIAN_POINT('Origin',(3.,1.,0.7));
#13781=CARTESIAN_POINT('',(2.75,1.,0.6));
#13782=CARTESIAN_POINT('Origin',(3.,1.,0.6));
#13783=CARTESIAN_POINT('',(2.75,1.,0.7));
#13784=CARTESIAN_POINT('Origin',(3.,1.,0.6));
#13785=CARTESIAN_POINT('Origin',(9.,-1.,0.7));
#13786=CARTESIAN_POINT('',(8.75,-1.,0.7));
#13787=CARTESIAN_POINT('Origin',(9.,-1.,0.7));
#13788=CARTESIAN_POINT('',(8.85,-1.,0.7));
#13789=CARTESIAN_POINT('Origin',(9.,-1.,0.7));
#13790=CARTESIAN_POINT('Origin',(9.,-1.,0.7));
#13791=CARTESIAN_POINT('',(8.75,-1.,0.6));
#13792=CARTESIAN_POINT('Origin',(9.,-1.,0.6));
#13793=CARTESIAN_POINT('',(8.75,-1.,0.7));
#13794=CARTESIAN_POINT('Origin',(9.,-1.,0.6));
#13795=CARTESIAN_POINT('Origin',(9.,1.,0.9));
#13796=CARTESIAN_POINT('',(8.85,1.,0.9));
#13797=CARTESIAN_POINT('',(8.85,1.,0.9));
#13798=CARTESIAN_POINT('Origin',(9.,1.,0.9));
#13799=CARTESIAN_POINT('Origin',(3.,-1.,0.9));
#13800=CARTESIAN_POINT('',(2.85,-1.,0.9));
#13801=CARTESIAN_POINT('',(2.85,-1.,0.9));
#13802=CARTESIAN_POINT('Origin',(3.,-1.,0.9));
#13803=CARTESIAN_POINT('Origin',(3.,1.,0.9));
#13804=CARTESIAN_POINT('',(2.85,1.,0.9));
#13805=CARTESIAN_POINT('',(2.85,1.,0.9));
#13806=CARTESIAN_POINT('Origin',(3.,1.,0.9));
#13807=CARTESIAN_POINT('Origin',(9.,-1.,0.9));
#13808=CARTESIAN_POINT('',(8.85,-1.,0.9));
#13809=CARTESIAN_POINT('',(8.85,-1.,0.9));
#13810=CARTESIAN_POINT('Origin',(9.,-1.,0.9));
#13811=CARTESIAN_POINT('Ctrl Pts',(11.5038445323837,1.18103800495499,1.1));
#13812=CARTESIAN_POINT('Ctrl Pts',(11.5184054935931,1.17950950960121,1.1));
#13813=CARTESIAN_POINT('Ctrl Pts',(11.5512741038969,1.16492409601325,1.1));
#13814=CARTESIAN_POINT('Ctrl Pts',(11.5664342774515,1.13103804392606,1.1));
#13815=CARTESIAN_POINT('Ctrl Pts',(11.5664342774515,1.11151675574496,1.1));
#13816=CARTESIAN_POINT('Ctrl Pts',(11.5062520964801,1.2039732708886,1.1));
#13817=CARTESIAN_POINT('Ctrl Pts',(11.5256097704488,1.20178950015253,1.09999449529541));
#13818=CARTESIAN_POINT('Ctrl Pts',(11.5690795528293,1.18226331832779,1.09998611288251));
#13819=CARTESIAN_POINT('Ctrl Pts',(11.5893469235372,1.13750635859412,1.09999170314796));
#13820=CARTESIAN_POINT('Ctrl Pts',(11.5895723566779,1.11151675574496,1.1));
#13821=CARTESIAN_POINT('Ctrl Pts',(11.5104252001437,1.2437276609947,1.08142124563721));
#13822=CARTESIAN_POINT('Ctrl Pts',(11.5380451995806,1.2404317701584,1.0816749051734));
#13823=CARTESIAN_POINT('Ctrl Pts',(11.5998825216457,1.21232138637678,1.08202590066027));
#13824=CARTESIAN_POINT('Ctrl Pts',(11.629084458256,1.14864330516641,1.08167049691811));
#13825=CARTESIAN_POINT('Ctrl Pts',(11.629673151989,1.11151675574496,1.08129017730416));
#13826=CARTESIAN_POINT('Ctrl Pts',(11.5120790720623,1.25948300155991,1.0418569252725));
#13827=CARTESIAN_POINT('Ctrl Pts',(11.5430287132786,1.25602537746711,1.04251419789099));
#13828=CARTESIAN_POINT('Ctrl Pts',(11.6126593164611,1.22478248685392,1.04343302714342));
#13829=CARTESIAN_POINT('Ctrl Pts',(11.6451104499416,1.15305025146974,1.04249969645955));
#13830=CARTESIAN_POINT('Ctrl Pts',(11.6454164251054,1.11151675574496,1.0415166534692));
#13831=CARTESIAN_POINT('Ctrl Pts',(11.5121826600865,1.26046981594516,1.0245894475956));
#13832=CARTESIAN_POINT('Ctrl Pts',(11.5433440226796,1.25715387309455,1.02536599531596));
#13833=CARTESIAN_POINT('Ctrl Pts',(11.6137195683385,1.22584236729999,1.02645725900057));
#13834=CARTESIAN_POINT('Ctrl Pts',(11.6462638499073,1.15328744881755,1.02534682499181));
#13835=CARTESIAN_POINT('Ctrl Pts',(11.6463246402318,1.11151675574496,1.02418687649944));
#13836=CARTESIAN_POINT('',(11.5664342774515,1.11151675574496,1.1));
#13837=CARTESIAN_POINT('',(11.6463246402318,1.11151675574496,1.02418687649943));
#13838=CARTESIAN_POINT('Origin',(11.5664342774515,1.11151675574496,1.02));
#13839=CARTESIAN_POINT('',(11.5121826600865,1.26046981594516,1.0245894475956));
#13840=CARTESIAN_POINT('Ctrl Pts',(11.6463246402318,1.11151675574496,1.02418687649944));
#13841=CARTESIAN_POINT('Ctrl Pts',(11.6462638499073,1.15328744881755,1.02534682499181));
#13842=CARTESIAN_POINT('Ctrl Pts',(11.6137195683385,1.22584236729999,1.02645725900057));
#13843=CARTESIAN_POINT('Ctrl Pts',(11.5433440226796,1.25715387309455,1.02536599531596));
#13844=CARTESIAN_POINT('Ctrl Pts',(11.5121826600865,1.26046981594516,1.0245894475956));
#13845=CARTESIAN_POINT('',(11.5038445323837,1.18103800495499,1.1));
#13846=CARTESIAN_POINT('Origin',(11.5038445323837,1.18103800495499,1.02));
#13847=CARTESIAN_POINT('Ctrl Pts',(11.5038445323837,1.18103800495499,1.1));
#13848=CARTESIAN_POINT('Ctrl Pts',(11.5184054935931,1.17950950960121,1.1));
#13849=CARTESIAN_POINT('Ctrl Pts',(11.5512741038969,1.16492409601325,1.1));
#13850=CARTESIAN_POINT('Ctrl Pts',(11.5664342774515,1.13103804392606,1.1));
#13851=CARTESIAN_POINT('Ctrl Pts',(11.5664342774515,1.11151675574496,1.1));
#13852=CARTESIAN_POINT('Origin',(11.5664342774515,0.626416499322631,1.02));
#13853=CARTESIAN_POINT('',(11.5664342774515,-1.11151675574496,1.1));
#13854=CARTESIAN_POINT('',(11.6463246402318,-1.11151675574496,1.02418687649944));
#13855=CARTESIAN_POINT('Origin',(11.5664342774515,-1.11151675574496,1.02));
#13856=CARTESIAN_POINT('',(11.6463246402318,0.626416499322631,1.02418687649944));
#13857=CARTESIAN_POINT('',(11.5664342774515,0.626416499322631,1.1));
#13858=CARTESIAN_POINT('Ctrl Pts',(11.5664342774515,-1.11151675574496,1.1));
#13859=CARTESIAN_POINT('Ctrl Pts',(11.5664342774515,-1.12615772189446,1.1));
#13860=CARTESIAN_POINT('Ctrl Pts',(11.5553715698491,-1.16037133170262,1.1));
#13861=CARTESIAN_POINT('Ctrl Pts',(11.5232591473477,-1.17900001114805,1.1));
#13862=CARTESIAN_POINT('Ctrl Pts',(11.5038445323837,-1.181038004955,1.1));
#13863=CARTESIAN_POINT('Ctrl Pts',(11.5895723566779,-1.11151675574496,1.1));
#13864=CARTESIAN_POINT('Ctrl Pts',(11.5894032818222,-1.13100895790003,1.09999377736097));
#13865=CARTESIAN_POINT('Ctrl Pts',(11.5744722352599,-1.17628172883974,1.09998542409303));
#13866=CARTESIAN_POINT('Ctrl Pts',(11.5320623284624,-1.20106157657112,1.09999266039387));
#13867=CARTESIAN_POINT('Ctrl Pts',(11.5062520964801,-1.2039732708886,1.1));
#13868=CARTESIAN_POINT('Ctrl Pts',(11.6296731519891,-1.11151675574496,1.0812901773042));
#13869=CARTESIAN_POINT('Ctrl Pts',(11.6292316316889,-1.13936166783705,1.08157541701493));
#13870=CARTESIAN_POINT('Ctrl Pts',(11.6075809177182,-1.20379599023677,1.08201780166247));
#13871=CARTESIAN_POINT('Ctrl Pts',(11.547251866094,-1.23933313987557,1.08175945835248));
#13872=CARTESIAN_POINT('Ctrl Pts',(11.5104252001437,-1.24372766099475,1.08142124563725));
#13873=CARTESIAN_POINT('Ctrl Pts',(11.6454164251054,-1.11151675574496,1.0415166534692));
#13874=CARTESIAN_POINT('Ctrl Pts',(11.6451869437323,-1.14266687756763,1.04225393571265));
#13875=CARTESIAN_POINT('Ctrl Pts',(11.6213248916312,-1.21516855113593,1.04341114660737));
#13876=CARTESIAN_POINT('Ctrl Pts',(11.5533452603892,-1.25487283609854,1.04273328876464));
#13877=CARTESIAN_POINT('Ctrl Pts',(11.5120790720623,-1.25948300155991,1.0418569252725));
#13878=CARTESIAN_POINT('Ctrl Pts',(11.6463246402318,-1.11151675574496,1.02418687649944));
#13879=CARTESIAN_POINT('Ctrl Pts',(11.6462790474884,-1.14284477557865,1.02505683786953));
#13880=CARTESIAN_POINT('Ctrl Pts',(11.6225012384517,-1.21608782625165,1.02643081388051));
#13881=CARTESIAN_POINT('Ctrl Pts',(11.5537311435827,-1.25604855880689,1.02562484455705));
#13882=CARTESIAN_POINT('Ctrl Pts',(11.5121826600865,-1.26046981594517,1.0245894475956));
#13883=CARTESIAN_POINT('',(11.5038445323837,-1.181038004955,1.1));
#13884=CARTESIAN_POINT('',(11.5121826600865,-1.26046981594517,1.02458944759559));
#13885=CARTESIAN_POINT('Origin',(11.5038445323837,-1.181038004955,1.02));
#13886=CARTESIAN_POINT('Ctrl Pts',(11.5121826600865,-1.26046981594517,1.0245894475956));
#13887=CARTESIAN_POINT('Ctrl Pts',(11.5537311435827,-1.25604855880689,1.02562484455705));
#13888=CARTESIAN_POINT('Ctrl Pts',(11.6225012384517,-1.21608782625165,1.02643081388051));
#13889=CARTESIAN_POINT('Ctrl Pts',(11.6462790474884,-1.14284477557865,1.02505683786953));
#13890=CARTESIAN_POINT('Ctrl Pts',(11.6463246402318,-1.11151675574496,1.02418687649944));
#13891=CARTESIAN_POINT('Ctrl Pts',(11.5664342774515,-1.11151675574496,1.1));
#13892=CARTESIAN_POINT('Ctrl Pts',(11.5664342774515,-1.12615772189446,1.1));
#13893=CARTESIAN_POINT('Ctrl Pts',(11.5553715698491,-1.16037133170262,1.1));
#13894=CARTESIAN_POINT('Ctrl Pts',(11.5232591473477,-1.17900001114805,1.1));
#13895=CARTESIAN_POINT('Ctrl Pts',(11.5038445323837,-1.181038004955,1.1));
#13896=CARTESIAN_POINT('Ctrl Pts',(11.5038445323836,-1.181038004955,1.1));
#13897=CARTESIAN_POINT('Ctrl Pts',(9.93221394244152,-1.34601544154236,1.1));
#13898=CARTESIAN_POINT('Ctrl Pts',(7.3047417451522,-1.56119993769491,1.1));
#13899=CARTESIAN_POINT('Ctrl Pts',(3.61332606662357,-1.48882378722464,1.1));
#13900=CARTESIAN_POINT('Ctrl Pts',(1.52093096174237,-1.20661833758759,1.1));
#13901=CARTESIAN_POINT('Ctrl Pts',(0.489277774073836,-0.993132359214002,
1.1));
#13902=CARTESIAN_POINT('Ctrl Pts',(11.5062520964801,-1.2039732708886,1.1));
#13903=CARTESIAN_POINT('Ctrl Pts',(9.93427206726409,-1.36902193231914,1.10000125302342));
#13904=CARTESIAN_POINT('Ctrl Pts',(7.30574352860662,-1.58436797372637,1.10000007151586));
#13905=CARTESIAN_POINT('Ctrl Pts',(3.61166276511536,-1.51194672535434,1.09999968963322));
#13906=CARTESIAN_POINT('Ctrl Pts',(1.51730587435546,-1.22941181706429,1.10000211650891));
#13907=CARTESIAN_POINT('Ctrl Pts',(0.48461766586479,-1.01565194352286,1.1));
#13908=CARTESIAN_POINT('Ctrl Pts',(11.5104252017938,-1.24372767671385,1.08142125970198));
#13909=CARTESIAN_POINT('Ctrl Pts',(9.93784299858723,-1.40889527428921,1.08136351975694));
#13910=CARTESIAN_POINT('Ctrl Pts',(7.3074712357333,-1.62451940065184,1.08127113650551));
#13911=CARTESIAN_POINT('Ctrl Pts',(3.60878747433083,-1.55202277432172,1.08130174433006));
#13912=CARTESIAN_POINT('Ctrl Pts',(1.51101154909588,-1.26891547398152,1.08143311272106));
#13913=CARTESIAN_POINT('Ctrl Pts',(0.476539293980871,-1.05469000198791,
1.08153107638517));
#13914=CARTESIAN_POINT('Ctrl Pts',(11.5120790720622,-1.25948300155992,1.0418569252725));
#13915=CARTESIAN_POINT('Ctrl Pts',(9.93924961011084,-1.42463380902671,1.04170731179674));
#13916=CARTESIAN_POINT('Ctrl Pts',(7.30815001459807,-1.64026117966461,1.0414672686166));
#13917=CARTESIAN_POINT('Ctrl Pts',(3.60765874156876,-1.56776897899067,1.04154646081959));
#13918=CARTESIAN_POINT('Ctrl Pts',(1.50852499534242,-1.28458904017411,1.04188830921359));
#13919=CARTESIAN_POINT('Ctrl Pts',(0.473312455428654,-1.07028343020201,
1.04214267388586));
#13920=CARTESIAN_POINT('Ctrl Pts',(11.5121826600865,-1.26046981594517,1.0245894475956));
#13921=CARTESIAN_POINT('Ctrl Pts',(9.9393350416019,-1.42558521977072,1.02441268379886));
#13922=CARTESIAN_POINT('Ctrl Pts',(7.30818539134325,-1.64115782448209,1.02412850358181));
#13923=CARTESIAN_POINT('Ctrl Pts',(3.607597182252,-1.56868448653922,1.02422201615766));
#13924=CARTESIAN_POINT('Ctrl Pts',(1.50836811330665,-1.28557739750152,1.02462705425916));
#13925=CARTESIAN_POINT('Ctrl Pts',(0.473097162761967,-1.07132381406029,
1.02492790083044));
#13926=CARTESIAN_POINT('',(0.489277774073836,-0.993132359214002,1.1));
#13927=CARTESIAN_POINT('',(0.473097162761967,-1.07132381406029,1.02492790083044));
#13928=CARTESIAN_POINT('Origin',(0.489277774073836,-0.993132359214002,1.02));
#13929=CARTESIAN_POINT('Ctrl Pts',(0.473097162761967,-1.07132381406029,
1.02492790083044));
#13930=CARTESIAN_POINT('Ctrl Pts',(1.50836811330665,-1.28557739750152,1.02462705425916));
#13931=CARTESIAN_POINT('Ctrl Pts',(3.607597182252,-1.56868448653922,1.02422201615766));
#13932=CARTESIAN_POINT('Ctrl Pts',(7.30818539134325,-1.64115782448209,1.02412850358181));
#13933=CARTESIAN_POINT('Ctrl Pts',(9.9393350416019,-1.42558521977072,1.02441268379886));
#13934=CARTESIAN_POINT('Ctrl Pts',(11.5121826600865,-1.26046981594517,1.0245894475956));
#13935=CARTESIAN_POINT('Ctrl Pts',(11.5038445323836,-1.181038004955,1.1));
#13936=CARTESIAN_POINT('Ctrl Pts',(9.93221394244152,-1.34601544154236,1.1));
#13937=CARTESIAN_POINT('Ctrl Pts',(7.3047417451522,-1.56119993769491,1.1));
#13938=CARTESIAN_POINT('Ctrl Pts',(3.61332606662357,-1.48882378722464,1.1));
#13939=CARTESIAN_POINT('Ctrl Pts',(1.52093096174237,-1.20661833758759,1.1));
#13940=CARTESIAN_POINT('Ctrl Pts',(0.489277774073836,-0.993132359214002,
1.1));
#13941=CARTESIAN_POINT('Ctrl Pts',(0.489277774073836,-0.993132359214003,
1.1));
#13942=CARTESIAN_POINT('Ctrl Pts',(0.47591459116406,-0.990367038259462,
1.1));
#13943=CARTESIAN_POINT('Ctrl Pts',(0.446638556739065,-0.974524902741032,
1.1));
#13944=CARTESIAN_POINT('Ctrl Pts',(0.433565722548535,-0.942876078073176,
1.1));
#13945=CARTESIAN_POINT('Ctrl Pts',(0.433565722548535,-0.924681003894255,
1.1));
#13946=CARTESIAN_POINT('Ctrl Pts',(0.48461766586479,-1.01565194352286,1.1));
#13947=CARTESIAN_POINT('Ctrl Pts',(0.466871946563175,-1.01185427439077,
1.09999555360656));
#13948=CARTESIAN_POINT('Ctrl Pts',(0.428148998320346,-0.990723083341879,
1.0999884677795));
#13949=CARTESIAN_POINT('Ctrl Pts',(0.410637366989639,-0.948905017863894,
1.09999228132016));
#13950=CARTESIAN_POINT('Ctrl Pts',(0.410427643322096,-0.924681003894255,
1.1));
#13951=CARTESIAN_POINT('Ctrl Pts',(0.47653584926364,-1.05470664829667,1.08154627613271));
#13952=CARTESIAN_POINT('Ctrl Pts',(0.451238756159369,-1.04914377880765,
1.08175207965746));
#13953=CARTESIAN_POINT('Ctrl Pts',(0.396142217510869,-1.01881823177681,
1.08201099971769));
#13954=CARTESIAN_POINT('Ctrl Pts',(0.370857020273576,-0.959285462196374,
1.08165947596025));
#13955=CARTESIAN_POINT('Ctrl Pts',(0.370309350093454,-0.924681003894255,
1.0813056591965));
#13956=CARTESIAN_POINT('Ctrl Pts',(0.473312455428654,-1.07028343020201,
1.04214267388586));
#13957=CARTESIAN_POINT('Ctrl Pts',(0.444929265438756,-1.064235408557,1.04267704697817));
#13958=CARTESIAN_POINT('Ctrl Pts',(0.382898223041383,-1.03040761468413,
1.04335444671884));
#13959=CARTESIAN_POINT('Ctrl Pts',(0.354868227955524,-0.963393056722486,
1.04243119239046));
#13960=CARTESIAN_POINT('Ctrl Pts',(0.354583574894625,-0.924681003894255,
1.0415166534692));
#13961=CARTESIAN_POINT('Ctrl Pts',(0.473097162761967,-1.07132381406029,
1.02492790083044));
#13962=CARTESIAN_POINT('Ctrl Pts',(0.444494893732137,-1.06536514830602,
1.02555992378854));
#13963=CARTESIAN_POINT('Ctrl Pts',(0.381802689524125,-1.03137574421946,
1.02636429433614));
#13964=CARTESIAN_POINT('Ctrl Pts',(0.353731913874551,-0.963614141904928,
1.02526599313355));
#13965=CARTESIAN_POINT('Ctrl Pts',(0.35367535976817,-0.924681003894255,
1.02418687649944));
#13966=CARTESIAN_POINT('',(0.433565722548535,-0.924681003894255,1.1));
#13967=CARTESIAN_POINT('',(0.35367535976817,-0.924681003894255,1.02418687649944));
#13968=CARTESIAN_POINT('Origin',(0.433565722548536,-0.924681003894255,1.02));
#13969=CARTESIAN_POINT('Ctrl Pts',(0.35367535976817,-0.924681003894255,
1.02418687649944));
#13970=CARTESIAN_POINT('Ctrl Pts',(0.353731913874551,-0.963614141904928,
1.02526599313355));
#13971=CARTESIAN_POINT('Ctrl Pts',(0.381802689524125,-1.03137574421946,
1.02636429433614));
#13972=CARTESIAN_POINT('Ctrl Pts',(0.444494893732137,-1.06536514830602,
1.02555992378854));
#13973=CARTESIAN_POINT('Ctrl Pts',(0.473097162761967,-1.07132381406029,
1.02492790083044));
#13974=CARTESIAN_POINT('Ctrl Pts',(0.489277774073836,-0.993132359214003,
1.1));
#13975=CARTESIAN_POINT('Ctrl Pts',(0.47591459116406,-0.990367038259462,
1.1));
#13976=CARTESIAN_POINT('Ctrl Pts',(0.446638556739065,-0.974524902741032,
1.1));
#13977=CARTESIAN_POINT('Ctrl Pts',(0.433565722548535,-0.942876078073176,
1.1));
#13978=CARTESIAN_POINT('Ctrl Pts',(0.433565722548535,-0.924681003894255,
1.1));
#13979=CARTESIAN_POINT('Origin',(0.433565722548536,-0.526416499322631,1.02));
#13980=CARTESIAN_POINT('',(0.433565722548536,0.924681003894255,1.1));
#13981=CARTESIAN_POINT('',(0.35367535976817,0.924681003894255,1.02418687649944));
#13982=CARTESIAN_POINT('Origin',(0.433565722548536,0.924681003894255,1.02));
#13983=CARTESIAN_POINT('',(0.35367535976817,-0.526416499322631,1.02418687649944));
#13984=CARTESIAN_POINT('',(0.433565722548536,-0.526416499322631,1.1));
#13985=CARTESIAN_POINT('Ctrl Pts',(0.433565722548535,0.924681003894255,
1.1));
#13986=CARTESIAN_POINT('Ctrl Pts',(0.433565722548535,0.94287607801605,1.1));
#13987=CARTESIAN_POINT('Ctrl Pts',(0.44664012289244,0.97452669098104,1.1));
#13988=CARTESIAN_POINT('Ctrl Pts',(0.475914591206016,0.990367038268144,
1.1));
#13989=CARTESIAN_POINT('Ctrl Pts',(0.489277774073836,0.993132359214003,
1.1));
#13990=CARTESIAN_POINT('Ctrl Pts',(0.410427643322096,0.924681003894255,
1.1));
#13991=CARTESIAN_POINT('Ctrl Pts',(0.410637366988981,0.948905017787839,
1.09999228132018));
#13992=CARTESIAN_POINT('Ctrl Pts',(0.428151078432557,0.99072545440496,1.09998846767325));
#13993=CARTESIAN_POINT('Ctrl Pts',(0.466871946618891,1.01185427440269,1.09999555360657));
#13994=CARTESIAN_POINT('Ctrl Pts',(0.48461766586479,1.01565194352286,1.1));
#13995=CARTESIAN_POINT('Ctrl Pts',(0.370309350093454,0.924681003894255,
1.0813056591965));
#13996=CARTESIAN_POINT('Ctrl Pts',(0.370857020271857,0.959285462087728,
1.08165947595914));
#13997=CARTESIAN_POINT('Ctrl Pts',(0.396145183504025,1.01882160767722,1.08201100382378));
#13998=CARTESIAN_POINT('Ctrl Pts',(0.451238756238795,1.04914377882512,1.08175207965681));
#13999=CARTESIAN_POINT('Ctrl Pts',(0.47653584926364,1.05470664829667,1.08154627613271));
#14000=CARTESIAN_POINT('Ctrl Pts',(0.354583574894625,0.924681003894255,
1.0415166534692));
#14001=CARTESIAN_POINT('Ctrl Pts',(0.35486822795463,0.963393056600943,1.04243119238759));
#14002=CARTESIAN_POINT('Ctrl Pts',(0.382901552879886,1.03041141096935,1.04335445746542));
#14003=CARTESIAN_POINT('Ctrl Pts',(0.444929265527871,1.06423540857599,1.04267704697649));
#14004=CARTESIAN_POINT('Ctrl Pts',(0.473312455428654,1.07028343020201,1.04214267388586));
#14005=CARTESIAN_POINT('Ctrl Pts',(0.35367535976817,0.924681003894255,1.02418687649944));
#14006=CARTESIAN_POINT('Ctrl Pts',(0.353731913874373,0.963614141782691,
1.02526599313016));
#14007=CARTESIAN_POINT('Ctrl Pts',(0.381806046235973,1.03137957549636,1.02636430709951));
#14008=CARTESIAN_POINT('Ctrl Pts',(0.44449489382194,1.06536514832473,1.02555992378656));
#14009=CARTESIAN_POINT('Ctrl Pts',(0.473097162761967,1.07132381406029,1.02492790083044));
#14010=CARTESIAN_POINT('',(0.489277774073836,0.993132359214003,1.1));
#14011=CARTESIAN_POINT('',(0.473097162761967,1.07132381406029,1.02492790083044));
#14012=CARTESIAN_POINT('Origin',(0.489277774073836,0.993132359214003,1.02));
#14013=CARTESIAN_POINT('Ctrl Pts',(0.473097162761967,1.07132381406029,1.02492790083044));
#14014=CARTESIAN_POINT('Ctrl Pts',(0.44449489382194,1.06536514832473,1.02555992378656));
#14015=CARTESIAN_POINT('Ctrl Pts',(0.381806046235973,1.03137957549636,1.02636430709951));
#14016=CARTESIAN_POINT('Ctrl Pts',(0.353731913874373,0.963614141782691,
1.02526599313016));
#14017=CARTESIAN_POINT('Ctrl Pts',(0.35367535976817,0.924681003894255,1.02418687649944));
#14018=CARTESIAN_POINT('Ctrl Pts',(0.433565722548535,0.924681003894255,
1.1));
#14019=CARTESIAN_POINT('Ctrl Pts',(0.433565722548535,0.94287607801605,1.1));
#14020=CARTESIAN_POINT('Ctrl Pts',(0.44664012289244,0.97452669098104,1.1));
#14021=CARTESIAN_POINT('Ctrl Pts',(0.475914591206016,0.990367038268144,
1.1));
#14022=CARTESIAN_POINT('Ctrl Pts',(0.489277774073836,0.993132359214003,
1.1));
#14023=CARTESIAN_POINT('Ctrl Pts',(0.489277774073836,0.993132359214003,
1.1));
#14024=CARTESIAN_POINT('Ctrl Pts',(1.52092917355268,1.20661796754713,1.1));
#14025=CARTESIAN_POINT('Ctrl Pts',(3.61335021200387,1.48882484395407,1.1));
#14026=CARTESIAN_POINT('Ctrl Pts',(7.30471495328446,1.56119985233321,1.1));
#14027=CARTESIAN_POINT('Ctrl Pts',(9.93221666658724,1.34601515558293,1.1));
#14028=CARTESIAN_POINT('Ctrl Pts',(11.5038445323836,1.18103800495499,1.1));
#14029=CARTESIAN_POINT('Ctrl Pts',(0.48461766586479,1.01565194352286,1.1));
#14030=CARTESIAN_POINT('Ctrl Pts',(1.51730408437175,1.22941144654908,1.10000211650524));
#14031=CARTESIAN_POINT('Ctrl Pts',(3.61168692820091,1.5119477834436,1.09999968963693));
#14032=CARTESIAN_POINT('Ctrl Pts',(7.30571671988008,1.58436788793099,1.10000007151498));
#14033=CARTESIAN_POINT('Ctrl Pts',(9.9342747920155,1.36902164623626,1.10000125302125));
#14034=CARTESIAN_POINT('Ctrl Pts',(11.5062520964801,1.2039732708886,1.1));
#14035=CARTESIAN_POINT('Ctrl Pts',(0.476539293980872,1.05469000198791,1.08153107638517));
#14036=CARTESIAN_POINT('Ctrl Pts',(1.51100975601983,1.26891510265927,1.08143311289086));
#14037=CARTESIAN_POINT('Ctrl Pts',(3.60881166804804,1.5520238347382,1.08130174382265));
#14038=CARTESIAN_POINT('Ctrl Pts',(7.30744439783659,1.62451931411139,1.08127113658549));
#14039=CARTESIAN_POINT('Ctrl Pts',(9.9378457243824,1.40889498800017,1.08136351985702));
#14040=CARTESIAN_POINT('Ctrl Pts',(11.5104252017938,1.24372767671385,1.08142125970198));
#14041=CARTESIAN_POINT('Ctrl Pts',(0.473312455428654,1.07028343020201,1.04214267388586));
#14042=CARTESIAN_POINT('Ctrl Pts',(1.50852320098322,1.28458866871296,1.04188830965449));
#14043=CARTESIAN_POINT('Ctrl Pts',(3.60768294746331,1.5677700397583,1.04154645950336));
#14044=CARTESIAN_POINT('Ctrl Pts',(7.30812316513016,1.64026109291585,1.04146726882447));
#14045=CARTESIAN_POINT('Ctrl Pts',(9.93925233633459,1.42463352276678,1.04170731205607));
#14046=CARTESIAN_POINT('Ctrl Pts',(11.5120790720622,1.25948300155991,1.0418569252725));
#14047=CARTESIAN_POINT('Ctrl Pts',(0.473097162761967,1.07132381406029,1.02492790083044));
#14048=CARTESIAN_POINT('Ctrl Pts',(1.50836631884621,1.28557702613055,1.02462705478063));
#14049=CARTESIAN_POINT('Ctrl Pts',(3.60762138890097,1.56868554702656,1.02422201460129));
#14050=CARTESIAN_POINT('Ctrl Pts',(7.30815854116978,1.64115773776738,1.02412850382783));
#14051=CARTESIAN_POINT('Ctrl Pts',(9.93933776785713,1.42558493357216,1.02441268410525));
#14052=CARTESIAN_POINT('Ctrl Pts',(11.5121826600865,1.26046981594517,1.0245894475956));
#14053=CARTESIAN_POINT('Ctrl Pts',(11.5121826600865,1.26046981594517,1.0245894475956));
#14054=CARTESIAN_POINT('Ctrl Pts',(9.93933776785713,1.42558493357216,1.02441268410525));
#14055=CARTESIAN_POINT('Ctrl Pts',(7.30815854116978,1.64115773776738,1.02412850382783));
#14056=CARTESIAN_POINT('Ctrl Pts',(3.60762138890097,1.56868554702656,1.02422201460129));
#14057=CARTESIAN_POINT('Ctrl Pts',(1.50836631884621,1.28557702613055,1.02462705478063));
#14058=CARTESIAN_POINT('Ctrl Pts',(0.473097162761967,1.07132381406029,1.02492790083044));
#14059=CARTESIAN_POINT('Ctrl Pts',(0.489277774073836,0.993132359214003,
1.1));
#14060=CARTESIAN_POINT('Ctrl Pts',(1.52092917355268,1.20661796754713,1.1));
#14061=CARTESIAN_POINT('Ctrl Pts',(3.61335021200387,1.48882484395407,1.1));
#14062=CARTESIAN_POINT('Ctrl Pts',(7.30471495328446,1.56119985233321,1.1));
#14063=CARTESIAN_POINT('Ctrl Pts',(9.93221666658724,1.34601515558293,1.1));
#14064=CARTESIAN_POINT('Ctrl Pts',(11.5038445323836,1.18103800495499,1.1));
#14065=CARTESIAN_POINT('Origin',(0.347167001354737,-1.05283299864526,0.9));
#14066=CARTESIAN_POINT('',(0.347167001354737,0.931160914046453,0.9));
#14067=CARTESIAN_POINT('Ctrl Pts',(0.347167001354737,0.931160914046453,
0.9));
#14068=CARTESIAN_POINT('Ctrl Pts',(0.34933645413337,0.929000934518636,0.941395625006663));
#14069=CARTESIAN_POINT('Ctrl Pts',(0.351505906937822,0.926840964458487,
0.982791250505987));
#14070=CARTESIAN_POINT('Ctrl Pts',(0.35367535976817,0.924681003894255,1.02418687649944));
#14071=CARTESIAN_POINT('',(0.347167001354737,-0.931160914046453,0.9));
#14072=CARTESIAN_POINT('',(0.347167001354737,-1.05283299864526,0.9));
#14073=CARTESIAN_POINT('Ctrl Pts',(0.35367535976817,-0.924681003894255,
1.02418687649944));
#14074=CARTESIAN_POINT('Ctrl Pts',(0.351505906937822,-0.926840964458487,
0.982791250505987));
#14075=CARTESIAN_POINT('Ctrl Pts',(0.34933645413337,-0.929000934518636,
0.941395625006663));
#14076=CARTESIAN_POINT('Ctrl Pts',(0.347167001354737,-0.931160914046453,
0.9));
#14077=CARTESIAN_POINT('Ctrl Pts',(0.346994979645257,0.93133218461645,0.89671763024815));
#14078=CARTESIAN_POINT('Ctrl Pts',(0.349221772992334,0.929115114391563,
0.939207378479044));
#14079=CARTESIAN_POINT('Ctrl Pts',(0.35144856636661,0.926898054140648,0.981697127228945));
#14080=CARTESIAN_POINT('Ctrl Pts',(0.35367535976817,0.924681003894255,1.02418687649944));
#14081=CARTESIAN_POINT('Ctrl Pts',(0.347101141748081,0.970260862175626,
0.898743323843195));
#14082=CARTESIAN_POINT('Ctrl Pts',(0.349327989245423,0.968041585482289,
0.94123294798136));
#14083=CARTESIAN_POINT('Ctrl Pts',(0.35155465541633,0.96582239703375,0.983722586263841));
#14084=CARTESIAN_POINT('Ctrl Pts',(0.353781503060223,0.96360313540272,1.02621221116359));
#14085=CARTESIAN_POINT('Ctrl Pts',(0.375231247034764,1.03797686888013,0.90080243726586));
#14086=CARTESIAN_POINT('Ctrl Pts',(0.377454726329371,1.03575393200526,0.943292036336267));
#14087=CARTESIAN_POINT('Ctrl Pts',(0.379678256934949,1.03353096064141,0.985781630873016));
#14088=CARTESIAN_POINT('Ctrl Pts',(0.381901729528225,1.03130803054038,1.02827123060239));
#14089=CARTESIAN_POINT('Ctrl Pts',(0.437891832981715,1.07196344732884,0.899291918906528));
#14090=CARTESIAN_POINT('Ctrl Pts',(0.440109459023804,1.06974216787274,0.941781905864285));
#14091=CARTESIAN_POINT('Ctrl Pts',(0.442327107866739,1.06752094195844,0.984271894420663));
#14092=CARTESIAN_POINT('Ctrl Pts',(0.44454471435444,1.06529967134173,1.02676188280081));
#14093=CARTESIAN_POINT('Ctrl Pts',(0.466484255634356,1.07794817238022,0.898105730168711));
#14094=CARTESIAN_POINT('Ctrl Pts',(0.46869984010673,1.07572875745303,0.940595920481163));
#14095=CARTESIAN_POINT('Ctrl Pts',(0.470915412358444,1.07350934859911,0.983086111716909));
#14096=CARTESIAN_POINT('Ctrl Pts',(0.473130972350001,1.07128994583173,1.02557630387858));
#14097=CARTESIAN_POINT('',(0.466583029361855,1.07784922788182,0.9));
#14098=CARTESIAN_POINT('Ctrl Pts',(0.473097162761967,1.07132381406029,1.02492790083044));
#14099=CARTESIAN_POINT('Ctrl Pts',(0.470925796725269,1.07349894615889,0.983285266331776));
#14100=CARTESIAN_POINT('Ctrl Pts',(0.468754418912838,1.07567408410356,0.941642632722456));
#14101=CARTESIAN_POINT('Ctrl Pts',(0.466583029361855,1.07784922788182,0.9));
#14102=CARTESIAN_POINT('Ctrl Pts',(0.466583029361856,1.07784922788182,0.9));
#14103=CARTESIAN_POINT('Ctrl Pts',(0.45605169130101,1.07567238924625,0.899999999995368));
#14104=CARTESIAN_POINT('Ctrl Pts',(0.445810809951917,1.07234818111891,0.899998625774342));
#14105=CARTESIAN_POINT('Ctrl Pts',(0.436024610942277,1.06798890472683,0.899998407511246));
#14106=CARTESIAN_POINT('Ctrl Pts',(0.42804650025127,1.0644350438709,0.899998229574221));
#14107=CARTESIAN_POINT('Ctrl Pts',(0.420370119207661,1.06019193848671,0.899998775177391));
#14108=CARTESIAN_POINT('Ctrl Pts',(0.413095080427888,1.05529723033767,0.89999964722522));
#14109=CARTESIAN_POINT('Ctrl Pts',(0.404948343152914,1.04981603600524,0.900000623762221));
#14110=CARTESIAN_POINT('Ctrl Pts',(0.3973835293994,1.04357129238854,0.900002055204145));
#14111=CARTESIAN_POINT('Ctrl Pts',(0.390528747317286,1.03663323920468,0.900000884971142));
#14112=CARTESIAN_POINT('Ctrl Pts',(0.38377850537204,1.02980099609921,0.899999732584995));
#14113=CARTESIAN_POINT('Ctrl Pts',(0.377716121663402,1.02229558340178,0.899996048870533));
#14114=CARTESIAN_POINT('Ctrl Pts',(0.372394770625083,1.01423711207676,0.899993306941804));
#14115=CARTESIAN_POINT('Ctrl Pts',(0.366459905306112,1.00524955578769,0.899990248888012));
#14116=CARTESIAN_POINT('Ctrl Pts',(0.361501411166698,0.995658501454654,
0.8999884459165));
#14117=CARTESIAN_POINT('Ctrl Pts',(0.35758177265536,0.985639755107121,0.899989063766683));
#14118=CARTESIAN_POINT('Ctrl Pts',(0.356156017388132,0.981995469968403,
0.8999892885076));
#14119=CARTESIAN_POINT('Ctrl Pts',(0.354868143601992,0.978294337124559,
0.899989797558581));
#14120=CARTESIAN_POINT('Ctrl Pts',(0.353722739999278,0.97454418014098,0.899990530873797));
#14121=CARTESIAN_POINT('Ctrl Pts',(0.350595356382139,0.964304837882626,
0.899992533100777));
#14122=CARTESIAN_POINT('Ctrl Pts',(0.348551371116014,0.953782216732967,
0.899996407005639));
#14123=CARTESIAN_POINT('Ctrl Pts',(0.347666342074759,0.943140644221274,
0.899998614621972));
#14124=CARTESIAN_POINT('Ctrl Pts',(0.347335396628921,0.939161362417926,
0.899999440132251));
#14125=CARTESIAN_POINT('Ctrl Pts',(0.347167001797138,0.935165318330998,
0.899999999966431));
#14126=CARTESIAN_POINT('Ctrl Pts',(0.347167001354737,0.931160914046453,
0.9));
#14127=CARTESIAN_POINT('Ctrl Pts',(0.466583029361855,1.07784922788182,0.9));
#14128=CARTESIAN_POINT('Ctrl Pts',(0.468719324182819,1.07566682993082,0.941642633610146));
#14129=CARTESIAN_POINT('Ctrl Pts',(0.470855619003782,1.07348443197981,0.983285267220292));
#14130=CARTESIAN_POINT('Ctrl Pts',(0.472991913824746,1.07130203402881,1.02492790083044));
#14131=CARTESIAN_POINT('Ctrl Pts',(4.1506201585889,1.83934349355009,0.9));
#14132=CARTESIAN_POINT('Ctrl Pts',(4.15133415151554,1.83716109559909,0.941642633610146));
#14133=CARTESIAN_POINT('Ctrl Pts',(4.15204814444219,1.83497869764808,0.983285267220293));
#14134=CARTESIAN_POINT('Ctrl Pts',(4.15276213736883,1.83279629969708,1.02492790083044));
#14135=CARTESIAN_POINT('Ctrl Pts',(7.83465728781595,1.65326443611903,0.9));
#14136=CARTESIAN_POINT('Ctrl Pts',(7.83394897884827,1.65108203816803,0.941642633610146));
#14137=CARTESIAN_POINT('Ctrl Pts',(7.83324066988059,1.64889964021702,0.983285267220292));
#14138=CARTESIAN_POINT('Ctrl Pts',(7.83253236091292,1.64671724226602,1.02492790083044));
#14139=CARTESIAN_POINT('Ctrl Pts',(11.518694417043,1.26698486563531,0.9));
#14140=CARTESIAN_POINT('Ctrl Pts',(11.516563806181,1.26480246768431,0.941642633610146));
#14141=CARTESIAN_POINT('Ctrl Pts',(11.514433195319,1.2626200697333,0.983285267220292));
#14142=CARTESIAN_POINT('Ctrl Pts',(11.512302584457,1.2604376717823,1.02492790083044));
#14143=CARTESIAN_POINT('',(11.518694417043,1.26698486563531,0.9));
#14144=CARTESIAN_POINT('Ctrl Pts',(11.518694417043,1.26698486563531,0.9));
#14145=CARTESIAN_POINT('Ctrl Pts',(11.5165238247878,1.26481317761477,0.941529815291285));
#14146=CARTESIAN_POINT('Ctrl Pts',(11.5143532391283,1.26264149437998,0.983059631155884));
#14147=CARTESIAN_POINT('Ctrl Pts',(11.5121826600865,1.26046981594516,1.0245894475956));
#14148=CARTESIAN_POINT('Ctrl Pts',(0.466583029361855,1.07784922788182,0.9));
#14149=CARTESIAN_POINT('Ctrl Pts',(4.1506201585889,1.83934349355009,0.9));
#14150=CARTESIAN_POINT('Ctrl Pts',(7.83465728781595,1.65326443611903,0.9));
#14151=CARTESIAN_POINT('Ctrl Pts',(11.518694417043,1.26698486563531,0.9));
#14152=CARTESIAN_POINT('Ctrl Pts',(11.5188237574534,1.26711427133763,0.897525337604991));
#14153=CARTESIAN_POINT('Ctrl Pts',(11.5166039145442,1.26489330787379,0.939997457644392));
#14154=CARTESIAN_POINT('Ctrl Pts',(11.5143840785328,1.26267234941507,0.982469578283382));
#14155=CARTESIAN_POINT('Ctrl Pts',(11.512164249443,1.26045139597664,1.02494169952389));
#14156=CARTESIAN_POINT('Ctrl Pts',(11.560356924166,1.2626472646828,0.899468475190601));
#14157=CARTESIAN_POINT('Ctrl Pts',(11.5581357517162,1.26042470505353,0.941940442504879));
#14158=CARTESIAN_POINT('Ctrl Pts',(11.5559146107476,1.25820228015812,0.984412418590584));
#14159=CARTESIAN_POINT('Ctrl Pts',(11.5536934488601,1.25597972716877,1.02688438676053));
#14160=CARTESIAN_POINT('Ctrl Pts',(11.6290545561482,1.22266466287338,0.9009785794625));
#14161=CARTESIAN_POINT('Ctrl Pts',(11.6268300646776,1.22044146949289,0.943450343593379));
#14162=CARTESIAN_POINT('Ctrl Pts',(11.6246055668724,1.21821824717544,0.985922105839347));
#14163=CARTESIAN_POINT('Ctrl Pts',(11.6223810783988,1.21599505938238,1.02839387038768));
#14164=CARTESIAN_POINT('Ctrl Pts',(11.652916631058,1.14949843694546,0.898404198500408));
#14165=CARTESIAN_POINT('Ctrl Pts',(11.6506907663731,1.14727726203421,0.940876003223652));
#14166=CARTESIAN_POINT('Ctrl Pts',(11.6484649368037,1.14505607393729,0.9833478090785));
#14167=CARTESIAN_POINT('Ctrl Pts',(11.6462390720682,1.14283490928962,1.02581961432614));
#14168=CARTESIAN_POINT('Ctrl Pts',(11.6530022067803,1.11817769023529,0.896771316447588));
#14169=CARTESIAN_POINT('Ctrl Pts',(11.6507763512808,1.11595737261641,0.939243169479033));
#14170=CARTESIAN_POINT('Ctrl Pts',(11.6485504957647,1.11373706111287,0.981715022829298));
#14171=CARTESIAN_POINT('Ctrl Pts',(11.6463246402318,1.11151675574496,1.02418687649944));
#14172=CARTESIAN_POINT('',(11.6528329986453,1.11800890309831,0.9));
#14173=CARTESIAN_POINT('Ctrl Pts',(11.6463246402318,1.11151675574496,1.02418687649944));
#14174=CARTESIAN_POINT('Ctrl Pts',(11.6484940930522,1.11368079904038,0.982791250696082));
#14175=CARTESIAN_POINT('Ctrl Pts',(11.6506635458567,1.11584484816443,0.941395625196594));
#14176=CARTESIAN_POINT('Ctrl Pts',(11.6528329986453,1.11800890309831,0.9));
#14177=CARTESIAN_POINT('Ctrl Pts',(11.6528329986453,1.11800890309831,0.9));
#14178=CARTESIAN_POINT('Ctrl Pts',(11.6528329983633,1.12876627611802,0.899999999993021));
#14179=CARTESIAN_POINT('Ctrl Pts',(11.6516446702457,1.13947128553817,0.899998527904116));
#14180=CARTESIAN_POINT('Ctrl Pts',(11.6493511293179,1.14994150848088,0.899998119066462));
#14181=CARTESIAN_POINT('Ctrl Pts',(11.6474764306251,1.15849967852608,0.89999778488999));
#14182=CARTESIAN_POINT('Ctrl Pts',(11.6448621032167,1.16690170462481,0.899998134702192));
#14183=CARTESIAN_POINT('Ctrl Pts',(11.6415284502961,1.17504213011111,0.899998933310541));
#14184=CARTESIAN_POINT('Ctrl Pts',(11.6374537398456,1.18499213918264,0.899999909446287));
#14185=CARTESIAN_POINT('Ctrl Pts',(11.6323486952005,1.19444663470912,0.900001674548864));
#14186=CARTESIAN_POINT('Ctrl Pts',(11.6262733681268,1.20322237541324,0.900000560254235));
#14187=CARTESIAN_POINT('Ctrl Pts',(11.6256011619285,1.20419336960417,0.900000436962806));
#14188=CARTESIAN_POINT('Ctrl Pts',(11.6249170295004,1.20515603220147,0.900000274771288));
#14189=CARTESIAN_POINT('Ctrl Pts',(11.6242210175348,1.20611009565643,0.900000065883751));
#14190=CARTESIAN_POINT('Ctrl Pts',(11.6197944794931,1.21217780481426,0.899998737388448));
#14191=CARTESIAN_POINT('Ctrl Pts',(11.6148881172219,1.21789846943619,0.899995595976687));
#14192=CARTESIAN_POINT('Ctrl Pts',(11.6095544776251,1.22323873890669,0.899992615091414));
#14193=CARTESIAN_POINT('Ctrl Pts',(11.601940589012,1.23086209181126,0.899988359811689));
#14194=CARTESIAN_POINT('Ctrl Pts',(11.5935341028624,1.23763544449334,0.899984652834703));
#14195=CARTESIAN_POINT('Ctrl Pts',(11.584505756877,1.24347857204465,0.899983891616646));
#14196=CARTESIAN_POINT('Ctrl Pts',(11.5791642013329,1.24693561616068,0.899983441247493));
#14197=CARTESIAN_POINT('Ctrl Pts',(11.5736041411459,1.25006639925598,0.89998394495257));
#14198=CARTESIAN_POINT('Ctrl Pts',(11.5678562300951,1.25284717822614,0.899985279956182));
#14199=CARTESIAN_POINT('Ctrl Pts',(11.5582100984591,1.25751387535486,0.899987520356298));
#14200=CARTESIAN_POINT('Ctrl Pts',(11.548125859505,1.26115381593413,0.899992245475585));
#14201=CARTESIAN_POINT('Ctrl Pts',(11.5377575652696,1.26367454383615,0.899995957332528));
#14202=CARTESIAN_POINT('Ctrl Pts',(11.5314967650479,1.26519666246525,0.899998198703601));
#14203=CARTESIAN_POINT('Ctrl Pts',(11.5251318445822,1.26630988651457,0.89999999997641));
#14204=CARTESIAN_POINT('Ctrl Pts',(11.518694417043,1.26698486563531,0.900000000000001));
#14205=CARTESIAN_POINT('Origin',(6.0828528088686,0.,1.1));
#14206=CARTESIAN_POINT('Origin',(11.6528329986453,1.25283299864526,0.9));
#14207=CARTESIAN_POINT('',(11.6528329986453,-1.11800890309831,0.9));
#14208=CARTESIAN_POINT('Ctrl Pts',(11.6528329986453,-1.11800890309831,0.9));
#14209=CARTESIAN_POINT('Ctrl Pts',(11.6506635458567,-1.11584484816443,0.941395625196595));
#14210=CARTESIAN_POINT('Ctrl Pts',(11.6484940930522,-1.11368079904038,0.98279125069608));
#14211=CARTESIAN_POINT('Ctrl Pts',(11.6463246402318,-1.11151675574497,1.02418687649944));
#14212=CARTESIAN_POINT('',(11.6528329986453,1.25283299864526,0.9));
#14213=CARTESIAN_POINT('Ctrl Pts',(0.466487690105381,-1.07794473197144,
0.898171596006697));
#14214=CARTESIAN_POINT('Ctrl Pts',(0.468702129741454,-1.07572646385346,
0.940639831040774));
#14215=CARTESIAN_POINT('Ctrl Pts',(0.470916557169473,-1.07350820180247,
0.983108066997194));
#14216=CARTESIAN_POINT('Ctrl Pts',(0.473130972350001,-1.07128994583173,
1.02557630387858));
#14217=CARTESIAN_POINT('Ctrl Pts',(0.428364464143914,-1.0699650947497,0.899753180570758));
#14218=CARTESIAN_POINT('Ctrl Pts',(0.430581658228805,-1.06774429850715,
0.942221140547455));
#14219=CARTESIAN_POINT('Ctrl Pts',(0.432798785432897,-1.06552370176641,
0.98468911452651));
#14220=CARTESIAN_POINT('Ctrl Pts',(0.435015961689253,-1.0633029131784,1.02715707577488));
#14221=CARTESIAN_POINT('Ctrl Pts',(0.367703220512368,-1.02873213740117,
0.900780809445176));
#14222=CARTESIAN_POINT('Ctrl Pts',(0.369926480243704,-1.02651076835199,
0.943248428164859));
#14223=CARTESIAN_POINT('Ctrl Pts',(0.372149767842394,-1.02428934262989,
0.985716042409561));
#14224=CARTESIAN_POINT('Ctrl Pts',(0.374373022752712,-1.02206798136513,
1.0281836617465));
#14225=CARTESIAN_POINT('Ctrl Pts',(0.347078053061478,-0.96052525347768,
0.898302765458188));
#14226=CARTESIAN_POINT('Ctrl Pts',(0.349303707759805,-0.958307704298137,
0.940770468670701));
#14227=CARTESIAN_POINT('Ctrl Pts',(0.351529312469145,-0.956090135383351,
0.983238173449507));
#14228=CARTESIAN_POINT('Ctrl Pts',(0.35375496723721,-0.953872602525604,
1.02570587749755));
#14229=CARTESIAN_POINT('Ctrl Pts',(0.346998431491642,-0.931328747842296,
0.896783495400846));
#14230=CARTESIAN_POINT('Ctrl Pts',(0.349224074223285,-0.929112823219098,
0.939251288581378));
#14231=CARTESIAN_POINT('Ctrl Pts',(0.3514497169821,-0.926896908559584,0.98171908228038));
#14232=CARTESIAN_POINT('Ctrl Pts',(0.35367535976817,-0.924681003894255,
1.02418687649944));
#14233=CARTESIAN_POINT('',(0.466583029361856,-1.07784922788182,0.9));
#14234=CARTESIAN_POINT('Ctrl Pts',(0.347167001354737,-0.931160914046453,
0.9));
#14235=CARTESIAN_POINT('Ctrl Pts',(0.34716700178392,-0.941918922633709,
0.89999999999014));
#14236=CARTESIAN_POINT('Ctrl Pts',(0.348348457226296,-0.952625037179515,
0.899998920330619));
#14237=CARTESIAN_POINT('Ctrl Pts',(0.350635026118381,-0.963095666025449,
0.899998881610567));
#14238=CARTESIAN_POINT('Ctrl Pts',(0.352503737518513,-0.971652846855939,
0.899998849966385));
#14239=CARTESIAN_POINT('Ctrl Pts',(0.355111758040853,-0.980053468583104,
0.899999488623984));
#14240=CARTESIAN_POINT('Ctrl Pts',(0.358442500181925,-0.988191468018609,
0.900000335306729));
#14241=CARTESIAN_POINT('Ctrl Pts',(0.362154764014137,-0.997261639077022,
0.900001278973215));
#14242=CARTESIAN_POINT('Ctrl Pts',(0.366728534310471,-1.00591832418384,
0.900002536038328));
#14243=CARTESIAN_POINT('Ctrl Pts',(0.372121756320194,-1.01402249383533,
0.900001139180886));
#14244=CARTESIAN_POINT('Ctrl Pts',(0.377460617198322,-1.02204497728291,
0.899999756403108));
#14245=CARTESIAN_POINT('Ctrl Pts',(0.383603173789776,-1.02952688289601,
0.899995781932517));
#14246=CARTESIAN_POINT('Ctrl Pts',(0.390441954151244,-1.03639066990207,
0.899992822880961));
#14247=CARTESIAN_POINT('Ctrl Pts',(0.398043576670582,-1.0440200884702,0.899989533757499));
#14248=CARTESIAN_POINT('Ctrl Pts',(0.406433719974705,-1.0508151602132,0.89998759991803));
#14249=CARTESIAN_POINT('Ctrl Pts',(0.415453314813275,-1.05667842789903,
0.899988256654353));
#14250=CARTESIAN_POINT('Ctrl Pts',(0.418717986328798,-1.05880065659603,
0.899988494362188));
#14251=CARTESIAN_POINT('Ctrl Pts',(0.422065457324696,-1.0608004431648,0.89998903479261));
#14252=CARTESIAN_POINT('Ctrl Pts',(0.425489105966494,-1.06267176343868,
0.899989815051126));
#14253=CARTESIAN_POINT('Ctrl Pts',(0.434878177994434,-1.06780370385578,
0.899991954845297));
#14254=CARTESIAN_POINT('Ctrl Pts',(0.444763746614507,-1.07193185662919,
0.899996125260102));
#14255=CARTESIAN_POINT('Ctrl Pts',(0.455000483828058,-1.07494865668414,
0.899998508040168));
#14256=CARTESIAN_POINT('Ctrl Pts',(0.458814676066972,-1.07607271165555,
0.899999395860286));
#14257=CARTESIAN_POINT('Ctrl Pts',(0.462677844602733,-1.07704202188211,
0.899999999981245));
#14258=CARTESIAN_POINT('Ctrl Pts',(0.466583029361856,-1.07784922788182,
0.9));
#14259=CARTESIAN_POINT('Ctrl Pts',(0.466583029361855,-1.07784922788182,
0.9));
#14260=CARTESIAN_POINT('Ctrl Pts',(0.468754418912838,-1.07567408410356,
0.941642632722455));
#14261=CARTESIAN_POINT('Ctrl Pts',(0.470925796725269,-1.07349894615889,
0.983285266331777));
#14262=CARTESIAN_POINT('Ctrl Pts',(0.473097162761967,-1.07132381406029,
1.02492790083044));
#14263=CARTESIAN_POINT('Ctrl Pts',(11.6530064742455,-1.11818194708322,0.896689888359234));
#14264=CARTESIAN_POINT('Ctrl Pts',(11.6507791962577,-1.11596021050721,0.93918888408639));
#14265=CARTESIAN_POINT('Ctrl Pts',(11.6485519182532,-1.11373848005435,0.98168788013277));
#14266=CARTESIAN_POINT('Ctrl Pts',(11.6463246402318,-1.11151675574497,1.02418687649944));
#14267=CARTESIAN_POINT('Ctrl Pts',(11.6528923732761,-1.15994294490385,0.898867064552409));
#14268=CARTESIAN_POINT('Ctrl Pts',(11.6506650597175,-1.15772003758575,0.94136599317676));
#14269=CARTESIAN_POINT('Ctrl Pts',(11.6484378630123,-1.15549719156343,0.98386493116262));
#14270=CARTESIAN_POINT('Ctrl Pts',(11.646210549347,-1.15327429380451,1.02636386026838));
#14271=CARTESIAN_POINT('Ctrl Pts',(11.6202781937939,-1.23241532269502,0.900946494593638));
#14272=CARTESIAN_POINT('Ctrl Pts',(11.6180528194216,-1.23019050716461,0.943445418126786));
#14273=CARTESIAN_POINT('Ctrl Pts',(11.61582741935,-1.22796567893144,0.985944339620759));
#14274=CARTESIAN_POINT('Ctrl Pts',(11.6136020491686,-1.22574086850162,1.02844326360542));
#14275=CARTESIAN_POINT('Ctrl Pts',(11.5499778903249,-1.26376827666489,0.89890126240954));
#14276=CARTESIAN_POINT('Ctrl Pts',(11.5477556460229,-1.26154471817669,0.941400412665532));
#14277=CARTESIAN_POINT('Ctrl Pts',(11.5455333818837,-1.25932119531825,0.983899563748029));
#14278=CARTESIAN_POINT('Ctrl Pts',(11.5433111490058,-1.25709764437074,1.02639871495137));
#14279=CARTESIAN_POINT('Ctrl Pts',(11.5188280133912,-1.26711852942379,0.897443909004722));
#14280=CARTESIAN_POINT('Ctrl Pts',(11.5166067518272,-1.2648961465915,0.93994317191011));
#14281=CARTESIAN_POINT('Ctrl Pts',(11.5143854971699,-1.26267376877071,0.982442435415857));
#14282=CARTESIAN_POINT('Ctrl Pts',(11.512164249443,-1.26045139597664,1.02494169952389));
#14283=CARTESIAN_POINT('',(11.518694417043,-1.26698486563531,0.9));
#14284=CARTESIAN_POINT('Ctrl Pts',(11.5121826600865,-1.26046981594517,1.02458944759559));
#14285=CARTESIAN_POINT('Ctrl Pts',(11.5143532391283,-1.26264149437998,0.983059631155874));
#14286=CARTESIAN_POINT('Ctrl Pts',(11.5165238247878,-1.26481317761477,0.941529815291278));
#14287=CARTESIAN_POINT('Ctrl Pts',(11.518694417043,-1.26698486563531,0.900000000000001));
#14288=CARTESIAN_POINT('Ctrl Pts',(11.518694417043,-1.26698486563531,0.9));
#14289=CARTESIAN_POINT('Ctrl Pts',(11.5293907449245,-1.26586333143554,0.89999999999772));
#14290=CARTESIAN_POINT('Ctrl Pts',(11.5399108669542,-1.26356499290392,0.899998338215302));
#14291=CARTESIAN_POINT('Ctrl Pts',(11.5500820708623,-1.26019169516113,0.899997799246518));
#14292=CARTESIAN_POINT('Ctrl Pts',(11.5583854467913,-1.257437865867,0.899997359253331));
#14293=CARTESIAN_POINT('Ctrl Pts',(11.5664568733073,-1.25396634382171,0.899997630752438));
#14294=CARTESIAN_POINT('Ctrl Pts',(11.5741940388996,-1.24980829733595,0.899998424072895));
#14295=CARTESIAN_POINT('Ctrl Pts',(11.5836658766397,-1.2447180170313,0.899999395255759));
#14296=CARTESIAN_POINT('Ctrl Pts',(11.5925370694996,-1.23865400393036,0.900001263097414));
#14297=CARTESIAN_POINT('Ctrl Pts',(11.6006317325417,-1.23169548876955,0.900000312360774));
#14298=CARTESIAN_POINT('Ctrl Pts',(11.6015335603822,-1.23092023936527,0.900000206439036));
#14299=CARTESIAN_POINT('Ctrl Pts',(11.602425722662,-1.23013384139825,0.900000061718141));
#14300=CARTESIAN_POINT('Ctrl Pts',(11.6033079529217,-1.22933637123764,0.899999870107331));
#14301=CARTESIAN_POINT('Ctrl Pts',(11.6088666967428,-1.22431168263841,0.899998662808674));
#14302=CARTESIAN_POINT('Ctrl Pts',(11.6140319692072,-1.21884801843051,0.89999566823453));
#14303=CARTESIAN_POINT('Ctrl Pts',(11.6187763833168,-1.21300082485405,0.899992820294732));
#14304=CARTESIAN_POINT('Ctrl Pts',(11.6255647330688,-1.20463460846846,0.899988745437233));
#14305=CARTESIAN_POINT('Ctrl Pts',(11.6314252437734,-1.1955686993246,0.899985180772245));
#14306=CARTESIAN_POINT('Ctrl Pts',(11.6362963259193,-1.18598144606113,0.899984461491908));
#14307=CARTESIAN_POINT('Ctrl Pts',(11.6391835002004,-1.18029891593343,0.899984035162064));
#14308=CARTESIAN_POINT('Ctrl Pts',(11.6417223485433,-1.1744324689719,0.89998453059116));
#14309=CARTESIAN_POINT('Ctrl Pts',(11.6438924319112,-1.16841525789854,0.899985826675912));
#14310=CARTESIAN_POINT('Ctrl Pts',(11.6475288754212,-1.15833212078062,0.899987998545922));
#14311=CARTESIAN_POINT('Ctrl Pts',(11.650098554646,-1.1479202064002,0.899992549671115));
#14312=CARTESIAN_POINT('Ctrl Pts',(11.6515257507029,-1.13734249630077,0.899996116295739));
#14313=CARTESIAN_POINT('Ctrl Pts',(11.6523885972688,-1.13094748084967,0.899998272586596));
#14314=CARTESIAN_POINT('Ctrl Pts',(11.6528329982118,-1.12449140232308,0.899999999966183));
#14315=CARTESIAN_POINT('Ctrl Pts',(11.6528329986453,-1.11800890309831,0.9));
#14316=CARTESIAN_POINT('Origin',(6.08275255467124,0.,0.9));
#14317=CARTESIAN_POINT('Ctrl Pts',(11.518694417043,-1.26698486563531,0.9));
#14318=CARTESIAN_POINT('Ctrl Pts',(7.83465728781595,-1.65326443611903,0.9));
#14319=CARTESIAN_POINT('Ctrl Pts',(4.1506201585889,-1.83934349355009,0.9));
#14320=CARTESIAN_POINT('Ctrl Pts',(0.466583029361856,-1.07784922788182,
0.9));
#14321=CARTESIAN_POINT('Ctrl Pts',(11.518694417043,-1.26698486563531,0.9));
#14322=CARTESIAN_POINT('Ctrl Pts',(11.516563806181,-1.26480246768431,0.941642633610146));
#14323=CARTESIAN_POINT('Ctrl Pts',(11.514433195319,-1.2626200697333,0.983285267220291));
#14324=CARTESIAN_POINT('Ctrl Pts',(11.512302584457,-1.2604376717823,1.02492790083044));
#14325=CARTESIAN_POINT('Ctrl Pts',(7.83465728781595,-1.65326443611903,0.9));
#14326=CARTESIAN_POINT('Ctrl Pts',(7.83394897884827,-1.65108203816803,0.941642633610146));
#14327=CARTESIAN_POINT('Ctrl Pts',(7.83324066988059,-1.64889964021702,0.983285267220291));
#14328=CARTESIAN_POINT('Ctrl Pts',(7.83253236091292,-1.64671724226602,1.02492790083044));
#14329=CARTESIAN_POINT('Ctrl Pts',(4.1506201585889,-1.8393434935501,0.9));
#14330=CARTESIAN_POINT('Ctrl Pts',(4.15133415151555,-1.83716109559909,0.941642633610146));
#14331=CARTESIAN_POINT('Ctrl Pts',(4.15204814444219,-1.83497869764808,0.983285267220291));
#14332=CARTESIAN_POINT('Ctrl Pts',(4.15276213736883,-1.83279629969708,1.02492790083044));
#14333=CARTESIAN_POINT('Ctrl Pts',(0.466583029361856,-1.07784922788182,
0.9));
#14334=CARTESIAN_POINT('Ctrl Pts',(0.468719324182819,-1.07566682993082,
0.941642633610146));
#14335=CARTESIAN_POINT('Ctrl Pts',(0.470855619003783,-1.07348443197981,
0.983285267220291));
#14336=CARTESIAN_POINT('Ctrl Pts',(0.472991913824746,-1.07130203402881,
1.02492790083044));
#19454=UNCERTAINTY_MEASURE_WITH_UNIT(LENGTH_MEASURE(0.001),#19472,
'DISTANCE_ACCURACY_VALUE',
'Maximum model space distance between geometric entities at asserted c
onnectivities');
#19458=UNCERTAINTY_MEASURE_WITH_UNIT(LENGTH_MEASURE(0.001),#19472,
'DISTANCE_ACCURACY_VALUE',
'Maximum model space distance between geometric entities at asserted c
onnectivities');
#19467=(
GEOMETRIC_REPRESENTATION_CONTEXT(3)
GLOBAL_UNCERTAINTY_ASSIGNED_CONTEXT((#19454))
GLOBAL_UNIT_ASSIGNED_CONTEXT((#19472,#19474,#19475))
REPRESENTATION_CONTEXT('','3D')
);
#19471=(
GEOMETRIC_REPRESENTATION_CONTEXT(3)
GLOBAL_UNCERTAINTY_ASSIGNED_CONTEXT((#19458))
GLOBAL_UNIT_ASSIGNED_CONTEXT((#19472,#19474,#19475))
REPRESENTATION_CONTEXT('','3D')
);
#19472=(
LENGTH_UNIT()
NAMED_UNIT(*)
SI_UNIT(.CENTI.,.METRE.)
);
#19474=(
NAMED_UNIT(*)
PLANE_ANGLE_UNIT()
SI_UNIT($,.RADIAN.)
);
#19475=(
NAMED_UNIT(*)
SI_UNIT($,.STERADIAN.)
SOLID_ANGLE_UNIT()
);
#19484=SHAPE_DEFINITION_REPRESENTATION(#19496,#19524);
#19496=PRODUCT_DEFINITION_SHAPE('',$,#19537);
#19524=SHAPE_REPRESENTATION('',(#7633),#19467);
#19528=PRODUCT_DEFINITION_CONTEXT('part definition',#19566,'design');
#19537=PRODUCT_DEFINITION('2026-11-10-01-30-02-394','Soft grip layer',#19549,
#19528);
#19549=PRODUCT_DEFINITION_FORMATION('',$,#19576);
#19566=APPLICATION_CONTEXT(
'Core Data for Automotive Mechanical Design Process');
#19567=PRODUCT_CONTEXT('part definition',#19566,'mechanical');
#19576=PRODUCT('2026-11-10-01-30-02-394','Soft grip layer',$,(#19567));
#19585=PRESENTATION_STYLE_ASSIGNMENT((#19593));
#19593=SURFACE_STYLE_USAGE(.BOTH.,#19601);
#19601=SURFACE_SIDE_STYLE('',(#19609));
#19609=SURFACE_STYLE_FILL_AREA(#19617);
#19617=FILL_AREA_STYLE('Sky blue soft grip',(#19625));
#19625=FILL_AREA_STYLE_COLOUR('Sky blue soft grip',#19633);
#19633=COLOUR_RGB('Sky blue soft grip',0.662745098039216,0.831372549019608,
0.949019607843137);
ENDSEC;
END-ISO-10303-21;
